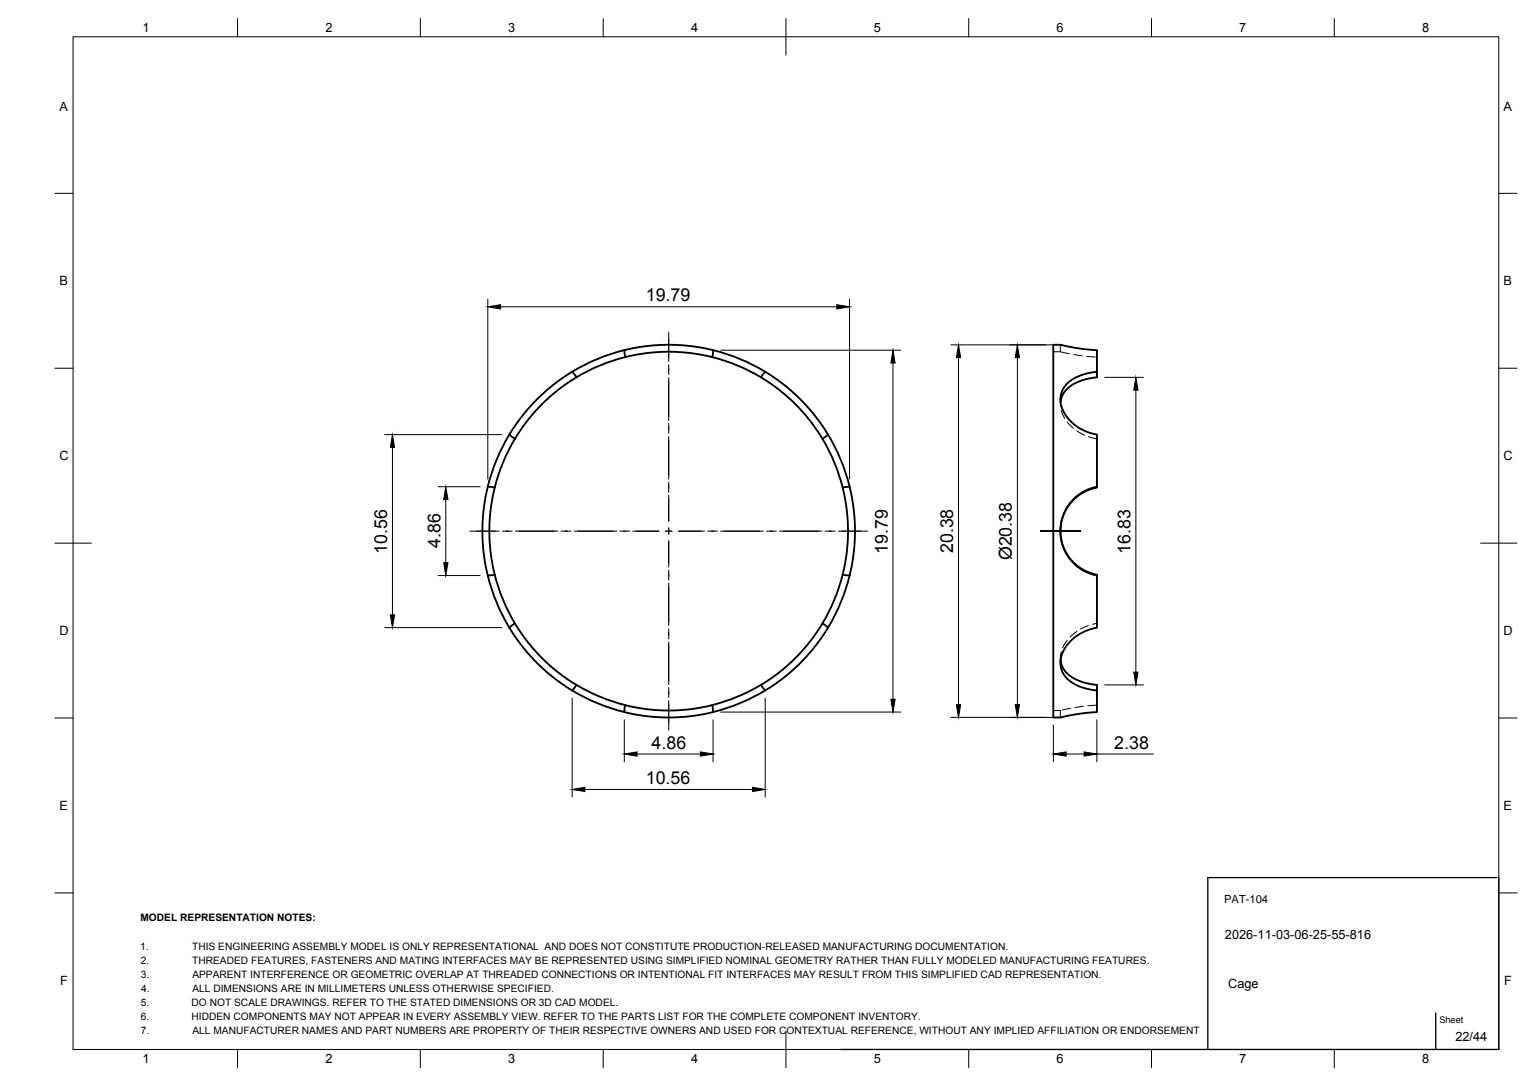
ISO-10303-21;
HEADER;
/* Generated by software containing ST-Developer
 * from STEP Tools, Inc. (www.steptools.com) 
 */

FILE_DESCRIPTION(
/* description */ ('Timing belt drive module 2 mm Pitch Timing 20T-40T'),

/* implementation_level */ '2;1');

FILE_NAME(
/* name */ 'Cage.step',
/* time_stamp */ '2026-10-28T03:25:12-07:00',
/* author */ (''),
/* organization */ (''),
/* preprocessor_version */ 'ST-DEVELOPER v20.2',
/* originating_system */ 'Autodesk Translation Framework v15.17.0.0',
/* authorisation */ '');

FILE_SCHEMA (('AUTOMOTIVE_DESIGN { 1 0 10303 214 3 1 1 }'));
ENDSEC;

DATA;
#10=MECHANICAL_DESIGN_GEOMETRIC_PRESENTATION_REPRESENTATION('',(#550),#17830);
#309=B_SPLINE_CURVE_WITH_KNOTS('',3,(#14805,#14806,#14807,#14808,#14809,
#14810,#14811,#14812,#14813,#14814,#14815,#14816,#14817,#14818,#14819,#14820,
#14821,#14822,#14823,#14824,#14825,#14826),.UNSPECIFIED.,.F.,.F.,(4,2,2,
2,2,2,2,2,2,2,4),(0.0473477652366656,0.126350602536658,0.189525903804987,
0.252701205073317,0.313298422430275,0.373895639787233,0.434492857144191,
0.495090074501149,0.558265375769478,0.621440677037807,0.7004435143378),
 .UNSPECIFIED.);
#310=B_SPLINE_CURVE_WITH_KNOTS('',3,(#14830,#14831,#14832,#14833,#14834,
#14835,#14836,#14837,#14838,#14839,#14840,#14841,#14842,#14843,#14844,#14845,
#14846,#14847,#14848,#14849,#14850,#14851),.UNSPECIFIED.,.F.,.F.,(4,2,2,
2,2,2,2,2,2,2,4),(0.0464897534940957,0.0852567806515119,0.170513561303024,
0.246687263103517,0.308657850341199,0.370628437578881,0.432599024816563,
0.494569612054245,0.570743313854739,0.656000094506251,0.694767121663666),
 .UNSPECIFIED.);
#311=B_SPLINE_CURVE_WITH_KNOTS('',3,(#14857,#14858,#14859,#14860,#14861,
#14862,#14863,#14864,#14865,#14866,#14867,#14868,#14869,#14870,#14871,#14872,
#14873,#14874,#14875,#14876,#14877,#14878),.UNSPECIFIED.,.F.,.F.,(4,2,2,
2,2,2,2,2,2,2,4),(0.0464897534940957,0.0852567806515118,0.170513561303024,
0.246687263103517,0.308657850341199,0.370628437578881,0.432599024816563,
0.494569612054245,0.570743313854738,0.65600009450625,0.694767121663666),
 .UNSPECIFIED.);
#312=B_SPLINE_CURVE_WITH_KNOTS('',3,(#14882,#14883,#14884,#14885,#14886,
#14887,#14888,#14889,#14890,#14891,#14892,#14893,#14894,#14895,#14896,#14897,
#14898,#14899,#14900,#14901,#14902,#14903),.UNSPECIFIED.,.F.,.F.,(4,2,2,
2,2,2,2,2,2,2,4),(0.0464897534940957,0.0852567806515119,0.170513561303024,
0.246687263103517,0.308657850341199,0.370628437578881,0.432599024816563,
0.494569612054245,0.570743313854739,0.656000094506251,0.694767121663666),
 .UNSPECIFIED.);
#313=B_SPLINE_CURVE_WITH_KNOTS('',3,(#14907,#14908,#14909,#14910,#14911,
#14912,#14913,#14914,#14915,#14916,#14917,#14918),.UNSPECIFIED.,.F.,.F.,
(4,2,2,2,2,4),(0.0464897534940957,0.0852567806515119,0.170513561303024,
0.246687263103517,0.308657850341199,0.370628437578881),.UNSPECIFIED.);
#314=B_SPLINE_CURVE_WITH_KNOTS('',3,(#14923,#14924,#14925,#14926,#14927,
#14928,#14929,#14930,#14931,#14932,#14933,#14934),.UNSPECIFIED.,.F.,.F.,
(4,2,2,2,2,4),(0.370628437578881,0.432599024816563,0.494569612054245,0.570743313854738,
0.65600009450625,0.694767121663666),.UNSPECIFIED.);
#315=B_SPLINE_CURVE_WITH_KNOTS('',3,(#14938,#14939,#14940,#14941,#14942,
#14943,#14944,#14945,#14946,#14947,#14948,#14949,#14950,#14951,#14952,#14953,
#14954,#14955,#14956,#14957,#14958,#14959),.UNSPECIFIED.,.F.,.F.,(4,2,2,
2,2,2,2,2,2,2,4),(0.0464897534940957,0.0852567806515121,0.170513561303024,
0.246687263103518,0.308657850341199,0.370628437578881,0.432599024816563,
0.494569612054245,0.570743313854738,0.65600009450625,0.694767121663666),
 .UNSPECIFIED.);
#316=B_SPLINE_CURVE_WITH_KNOTS('',3,(#14963,#14964,#14965,#14966,#14967,
#14968,#14969,#14970,#14971,#14972,#14973,#14974,#14975,#14976,#14977,#14978,
#14979,#14980,#14981,#14982,#14983,#14984),.UNSPECIFIED.,.F.,.F.,(4,2,2,
2,2,2,2,2,2,2,4),(0.0464897534940957,0.0852567806515119,0.170513561303024,
0.246687263103517,0.308657850341199,0.370628437578881,0.432599024816563,
0.494569612054245,0.570743313854738,0.65600009450625,0.694767121663667),
 .UNSPECIFIED.);
#317=B_SPLINE_CURVE_WITH_KNOTS('',3,(#14988,#14989,#14990,#14991,#14992,
#14993,#14994,#14995,#14996,#14997,#14998,#14999,#15000,#15001,#15002,#15003,
#15004,#15005,#15006,#15007,#15008,#15009),.UNSPECIFIED.,.F.,.F.,(4,2,2,
2,2,2,2,2,2,2,4),(0.0464897534940957,0.0852567806515119,0.170513561303024,
0.246687263103517,0.308657850341199,0.370628437578881,0.432599024816563,
0.494569612054245,0.570743313854738,0.65600009450625,0.694767121663666),
 .UNSPECIFIED.);
#318=B_SPLINE_CURVE_WITH_KNOTS('',3,(#15013,#15014,#15015,#15016,#15017,
#15018,#15019,#15020,#15021,#15022,#15023,#15024,#15025,#15026,#15027,#15028,
#15029,#15030,#15031,#15032,#15033,#15034),.UNSPECIFIED.,.F.,.F.,(4,2,2,
2,2,2,2,2,2,2,4),(0.0464897534940957,0.0852567806515119,0.170513561303024,
0.246687263103517,0.308657850341199,0.370628437578881,0.432599024816563,
0.494569612054245,0.570743313854739,0.656000094506251,0.694767121663667),
 .UNSPECIFIED.);
#319=B_SPLINE_CURVE_WITH_KNOTS('',3,(#15042,#15043,#15044,#15045,#15046,
#15047,#15048,#15049,#15050,#15051,#15052,#15053,#15054,#15055,#15056,#15057,
#15058,#15059,#15060,#15061,#15062,#15063),.UNSPECIFIED.,.F.,.F.,(4,2,2,
2,2,2,2,2,2,2,4),(0.0473477652366656,0.126350602536658,0.189525903804987,
0.252701205073316,0.313298422430274,0.373895639787232,0.434492857144191,
0.495090074501149,0.558265375769478,0.621440677037807,0.7004435143378),
 .UNSPECIFIED.);
#320=B_SPLINE_CURVE_WITH_KNOTS('',3,(#15071,#15072,#15073,#15074,#15075,
#15076,#15077,#15078,#15079,#15080,#15081,#15082,#15083,#15084,#15085,#15086,
#15087,#15088,#15089,#15090,#15091,#15092),.UNSPECIFIED.,.F.,.F.,(4,2,2,
2,2,2,2,2,2,2,4),(0.0473477652366656,0.126350602536658,0.189525903804987,
0.252701205073317,0.313298422430275,0.373895639787233,0.434492857144191,
0.495090074501149,0.558265375769478,0.621440677037807,0.7004435143378),
 .UNSPECIFIED.);
#321=B_SPLINE_CURVE_WITH_KNOTS('',3,(#15101,#15102,#15103,#15104,#15105,
#15106,#15107,#15108,#15109,#15110,#15111,#15112),.UNSPECIFIED.,.F.,.F.,
(4,2,2,2,2,4),(0.0473477652366656,0.126350602536658,0.189525903804987,0.252701205073316,
0.313298422430275,0.373895639787233),.UNSPECIFIED.);
#322=B_SPLINE_CURVE_WITH_KNOTS('',3,(#15114,#15115,#15116,#15117,#15118,
#15119,#15120,#15121,#15122,#15123,#15124,#15125),.UNSPECIFIED.,.F.,.F.,
(4,2,2,2,2,4),(0.373895639787233,0.434492857144191,0.495090074501149,0.558265375769478,
0.621440677037807,0.7004435143378),.UNSPECIFIED.);
#323=B_SPLINE_CURVE_WITH_KNOTS('',3,(#15132,#15133,#15134,#15135,#15136,
#15137,#15138,#15139,#15140,#15141,#15142,#15143,#15144,#15145,#15146,#15147,
#15148,#15149,#15150,#15151,#15152,#15153),.UNSPECIFIED.,.F.,.F.,(4,2,2,
2,2,2,2,2,2,2,4),(0.0473477652366656,0.126350602536658,0.189525903804987,
0.252701205073316,0.313298422430275,0.373895639787233,0.434492857144191,
0.495090074501149,0.558265375769478,0.621440677037807,0.7004435143378),
 .UNSPECIFIED.);
#324=B_SPLINE_CURVE_WITH_KNOTS('',3,(#15161,#15162,#15163,#15164,#15165,
#15166,#15167,#15168,#15169,#15170,#15171,#15172,#15173,#15174,#15175,#15176,
#15177,#15178,#15179,#15180,#15181,#15182),.UNSPECIFIED.,.F.,.F.,(4,2,2,
2,2,2,2,2,2,2,4),(0.0473477652366656,0.126350602536658,0.189525903804987,
0.252701205073317,0.313298422430275,0.373895639787233,0.434492857144191,
0.495090074501149,0.558265375769478,0.621440677037807,0.7004435143378),
 .UNSPECIFIED.);
#325=B_SPLINE_CURVE_WITH_KNOTS('',3,(#15190,#15191,#15192,#15193,#15194,
#15195,#15196,#15197,#15198,#15199,#15200,#15201,#15202,#15203,#15204,#15205,
#15206,#15207,#15208,#15209,#15210,#15211),.UNSPECIFIED.,.F.,.F.,(4,2,2,
2,2,2,2,2,2,2,4),(0.0473477652366656,0.126350602536658,0.189525903804987,
0.252701205073316,0.313298422430275,0.373895639787233,0.434492857144191,
0.495090074501149,0.558265375769478,0.621440677037807,0.7004435143378),
 .UNSPECIFIED.);
#326=B_SPLINE_CURVE_WITH_KNOTS('',3,(#15220,#15221,#15222,#15223,#15224,
#15225,#15226,#15227,#15228,#15229,#15230,#15231,#15232,#15233,#15234,#15235,
#15236,#15237,#15238,#15239,#15240,#15241),.UNSPECIFIED.,.F.,.F.,(4,2,2,
2,2,2,2,2,2,2,4),(0.0473477652366656,0.126350602536658,0.189525903804987,
0.252701205073317,0.313298422430275,0.373895639787233,0.434492857144191,
0.495090074501149,0.558265375769478,0.621440677037807,0.7004435143378),
 .UNSPECIFIED.);
#393=SPHERICAL_SURFACE('',#9935,0.247676);
#394=SPHERICAL_SURFACE('',#9951,0.247676);
#395=SPHERICAL_SURFACE('',#9956,0.247676);
#396=SPHERICAL_SURFACE('',#9961,0.247676);
#397=SPHERICAL_SURFACE('',#9966,0.247676);
#398=SPHERICAL_SURFACE('',#9971,0.247676);
#399=SPHERICAL_SURFACE('',#9976,0.247676);
#400=SPHERICAL_SURFACE('',#9984,0.247676);
#457=SHAPE_REPRESENTATION_RELATIONSHIP('SRR','None',#18028,#500);
#500=ADVANCED_BREP_SHAPE_REPRESENTATION('',(#608),#17803);
#550=STYLED_ITEM('',(#18317),#608);
#608=MANIFOLD_SOLID_BREP('Continuous crown cage',#9007);
#713=FACE_BOUND('',#1767,.T.);
#857=PLANE('',#9948);
#858=PLANE('',#9953);
#859=PLANE('',#9958);
#860=PLANE('',#9963);
#861=PLANE('',#9968);
#862=PLANE('',#9973);
#863=PLANE('',#9982);
#864=PLANE('',#9986);
#865=PLANE('',#9987);
#1152=FACE_OUTER_BOUND('',#1749,.T.);
#1153=FACE_OUTER_BOUND('',#1750,.T.);
#1154=FACE_OUTER_BOUND('',#1751,.T.);
#1155=FACE_OUTER_BOUND('',#1752,.T.);
#1156=FACE_OUTER_BOUND('',#1753,.T.);
#1157=FACE_OUTER_BOUND('',#1754,.T.);
#1158=FACE_OUTER_BOUND('',#1755,.T.);
#1159=FACE_OUTER_BOUND('',#1756,.T.);
#1160=FACE_OUTER_BOUND('',#1757,.T.);
#1161=FACE_OUTER_BOUND('',#1758,.T.);
#1162=FACE_OUTER_BOUND('',#1759,.T.);
#1163=FACE_OUTER_BOUND('',#1760,.T.);
#1164=FACE_OUTER_BOUND('',#1761,.T.);
#1165=FACE_OUTER_BOUND('',#1762,.T.);
#1166=FACE_OUTER_BOUND('',#1763,.T.);
#1167=FACE_OUTER_BOUND('',#1764,.T.);
#1168=FACE_OUTER_BOUND('',#1765,.T.);
#1169=FACE_OUTER_BOUND('',#1766,.T.);
#1170=FACE_OUTER_BOUND('',#1768,.T.);
#1749=EDGE_LOOP('',(#6621,#6622,#6623,#6624));
#1750=EDGE_LOOP('',(#6625,#6626,#6627,#6628,#6629,#6630,#6631,#6632,#6633,
#6634,#6635,#6636,#6637,#6638,#6639,#6640,#6641,#6642,#6643,#6644));
#1751=EDGE_LOOP('',(#6645,#6646,#6647,#6648));
#1752=EDGE_LOOP('',(#6649,#6650,#6651,#6652));
#1753=EDGE_LOOP('',(#6653,#6654,#6655,#6656));
#1754=EDGE_LOOP('',(#6657,#6658,#6659,#6660));
#1755=EDGE_LOOP('',(#6661,#6662,#6663,#6664));
#1756=EDGE_LOOP('',(#6665,#6666,#6667,#6668,#6669,#6670));
#1757=EDGE_LOOP('',(#6671,#6672,#6673,#6674));
#1758=EDGE_LOOP('',(#6675,#6676,#6677,#6678));
#1759=EDGE_LOOP('',(#6679,#6680,#6681,#6682));
#1760=EDGE_LOOP('',(#6683,#6684,#6685,#6686));
#1761=EDGE_LOOP('',(#6687,#6688,#6689,#6690));
#1762=EDGE_LOOP('',(#6691,#6692,#6693,#6694));
#1763=EDGE_LOOP('',(#6695,#6696,#6697,#6698,#6699,#6700,#6701,#6702,#6703,
#6704,#6705,#6706,#6707,#6708,#6709,#6710,#6711,#6712,#6713,#6714));
#1764=EDGE_LOOP('',(#6715,#6716,#6717,#6718));
#1765=EDGE_LOOP('',(#6719,#6720,#6721,#6722));
#1766=EDGE_LOOP('',(#6723));
#1767=EDGE_LOOP('',(#6724));
#1768=EDGE_LOOP('',(#6725,#6726,#6727,#6728));
#2346=CIRCLE('',#9936,0.243053047864041);
#2347=CIRCLE('',#9937,0.243053047864041);
#2348=CIRCLE('',#9939,1.019052);
#2349=CIRCLE('',#9940,1.019052);
#2350=CIRCLE('',#9941,1.019052);
#2351=CIRCLE('',#9942,1.019052);
#2352=CIRCLE('',#9943,1.019052);
#2353=CIRCLE('',#9944,1.019052);
#2354=CIRCLE('',#9945,1.019052);
#2355=CIRCLE('',#9946,1.019052);
#2356=CIRCLE('',#9947,1.019052);
#2357=CIRCLE('',#9949,0.980948);
#2358=CIRCLE('',#9950,0.243053047864041);
#2359=CIRCLE('',#9952,0.243053047864041);
#2360=CIRCLE('',#9954,0.980948);
#2361=CIRCLE('',#9955,0.243053047864041);
#2362=CIRCLE('',#9957,0.243053047864041);
#2363=CIRCLE('',#9959,0.980948);
#2364=CIRCLE('',#9960,0.243053047864041);
#2365=CIRCLE('',#9962,0.243053047864041);
#2366=CIRCLE('',#9964,0.980948);
#2367=CIRCLE('',#9965,0.243053047864041);
#2368=CIRCLE('',#9967,0.243053047864041);
#2369=CIRCLE('',#9969,0.980948);
#2370=CIRCLE('',#9970,0.243053047864041);
#2371=CIRCLE('',#9972,0.243053047864041);
#2372=CIRCLE('',#9974,0.980948);
#2373=CIRCLE('',#9975,0.243053047864041);
#2374=CIRCLE('',#9977,0.243053047864041);
#2375=CIRCLE('',#9979,0.980948);
#2376=CIRCLE('',#9980,0.980948);
#2377=CIRCLE('',#9981,0.980948);
#2378=CIRCLE('',#9983,0.243053047864041);
#2379=CIRCLE('',#9985,0.243053047864041);
#3008=LINE('',#14920,#3486);
#3009=LINE('',#15216,#3487);
#3486=VECTOR('',#11879,1.019052);
#3487=VECTOR('',#11956,0.980948);
#4038=VERTEX_POINT('',#14803);
#4039=VERTEX_POINT('',#14804);
#4040=VERTEX_POINT('',#14827);
#4041=VERTEX_POINT('',#14829);
#4042=VERTEX_POINT('',#14854);
#4043=VERTEX_POINT('',#14856);
#4044=VERTEX_POINT('',#14879);
#4045=VERTEX_POINT('',#14881);
#4046=VERTEX_POINT('',#14904);
#4047=VERTEX_POINT('',#14906);
#4048=VERTEX_POINT('',#14919);
#4049=VERTEX_POINT('',#14922);
#4050=VERTEX_POINT('',#14935);
#4051=VERTEX_POINT('',#14937);
#4052=VERTEX_POINT('',#14960);
#4053=VERTEX_POINT('',#14962);
#4054=VERTEX_POINT('',#14985);
#4055=VERTEX_POINT('',#14987);
#4056=VERTEX_POINT('',#15010);
#4057=VERTEX_POINT('',#15012);
#4058=VERTEX_POINT('',#15037);
#4059=VERTEX_POINT('',#15041);
#4060=VERTEX_POINT('',#15066);
#4061=VERTEX_POINT('',#15070);
#4062=VERTEX_POINT('',#15095);
#4063=VERTEX_POINT('',#15099);
#4064=VERTEX_POINT('',#15100);
#4065=VERTEX_POINT('',#15127);
#4066=VERTEX_POINT('',#15131);
#4067=VERTEX_POINT('',#15156);
#4068=VERTEX_POINT('',#15160);
#4069=VERTEX_POINT('',#15185);
#4070=VERTEX_POINT('',#15189);
#4071=VERTEX_POINT('',#15214);
#4072=VERTEX_POINT('',#15217);
#4073=VERTEX_POINT('',#15219);
#4993=EDGE_CURVE('',#4038,#4039,#309,.T.);
#4994=EDGE_CURVE('',#4040,#4038,#2346,.T.);
#4995=EDGE_CURVE('',#4041,#4040,#310,.T.);
#4996=EDGE_CURVE('',#4039,#4041,#2347,.T.);
#4997=EDGE_CURVE('',#4042,#4040,#2348,.T.);
#4998=EDGE_CURVE('',#4042,#4043,#311,.T.);
#4999=EDGE_CURVE('',#4044,#4043,#2349,.T.);
#5000=EDGE_CURVE('',#4044,#4045,#312,.T.);
#5001=EDGE_CURVE('',#4046,#4045,#2350,.T.);
#5002=EDGE_CURVE('',#4046,#4047,#313,.T.);
#5003=EDGE_CURVE('',#4047,#4048,#3008,.T.);
#5004=EDGE_CURVE('',#4048,#4048,#2351,.T.);
#5005=EDGE_CURVE('',#4047,#4049,#314,.T.);
#5006=EDGE_CURVE('',#4050,#4049,#2352,.T.);
#5007=EDGE_CURVE('',#4050,#4051,#315,.T.);
#5008=EDGE_CURVE('',#4052,#4051,#2353,.T.);
#5009=EDGE_CURVE('',#4052,#4053,#316,.T.);
#5010=EDGE_CURVE('',#4054,#4053,#2354,.T.);
#5011=EDGE_CURVE('',#4054,#4055,#317,.T.);
#5012=EDGE_CURVE('',#4056,#4055,#2355,.T.);
#5013=EDGE_CURVE('',#4056,#4057,#318,.T.);
#5014=EDGE_CURVE('',#4041,#4057,#2356,.T.);
#5015=EDGE_CURVE('',#4038,#4058,#2357,.T.);
#5016=EDGE_CURVE('',#4058,#4042,#2358,.T.);
#5017=EDGE_CURVE('',#4059,#4058,#319,.T.);
#5018=EDGE_CURVE('',#4043,#4059,#2359,.T.);
#5019=EDGE_CURVE('',#4059,#4060,#2360,.T.);
#5020=EDGE_CURVE('',#4060,#4044,#2361,.T.);
#5021=EDGE_CURVE('',#4061,#4060,#320,.T.);
#5022=EDGE_CURVE('',#4045,#4061,#2362,.T.);
#5023=EDGE_CURVE('',#4061,#4062,#2363,.T.);
#5024=EDGE_CURVE('',#4062,#4046,#2364,.T.);
#5025=EDGE_CURVE('',#4063,#4064,#321,.T.);
#5026=EDGE_CURVE('',#4049,#4063,#2365,.T.);
#5027=EDGE_CURVE('',#4064,#4062,#322,.T.);
#5028=EDGE_CURVE('',#4063,#4065,#2366,.T.);
#5029=EDGE_CURVE('',#4065,#4050,#2367,.T.);
#5030=EDGE_CURVE('',#4066,#4065,#323,.T.);
#5031=EDGE_CURVE('',#4051,#4066,#2368,.T.);
#5032=EDGE_CURVE('',#4066,#4067,#2369,.T.);
#5033=EDGE_CURVE('',#4067,#4052,#2370,.T.);
#5034=EDGE_CURVE('',#4068,#4067,#324,.T.);
#5035=EDGE_CURVE('',#4053,#4068,#2371,.T.);
#5036=EDGE_CURVE('',#4068,#4069,#2372,.T.);
#5037=EDGE_CURVE('',#4069,#4054,#2373,.T.);
#5038=EDGE_CURVE('',#4070,#4069,#325,.T.);
#5039=EDGE_CURVE('',#4055,#4070,#2374,.T.);
#5040=EDGE_CURVE('',#4071,#4071,#2375,.T.);
#5041=EDGE_CURVE('',#4071,#4064,#3009,.T.);
#5042=EDGE_CURVE('',#4072,#4039,#2376,.T.);
#5043=EDGE_CURVE('',#4072,#4073,#326,.T.);
#5044=EDGE_CURVE('',#4070,#4073,#2377,.T.);
#5045=EDGE_CURVE('',#4057,#4072,#2378,.T.);
#5046=EDGE_CURVE('',#4073,#4056,#2379,.T.);
#6621=ORIENTED_EDGE('',*,*,#4993,.F.);
#6622=ORIENTED_EDGE('',*,*,#4994,.F.);
#6623=ORIENTED_EDGE('',*,*,#4995,.F.);
#6624=ORIENTED_EDGE('',*,*,#4996,.F.);
#6625=ORIENTED_EDGE('',*,*,#4995,.T.);
#6626=ORIENTED_EDGE('',*,*,#4997,.F.);
#6627=ORIENTED_EDGE('',*,*,#4998,.T.);
#6628=ORIENTED_EDGE('',*,*,#4999,.F.);
#6629=ORIENTED_EDGE('',*,*,#5000,.T.);
#6630=ORIENTED_EDGE('',*,*,#5001,.F.);
#6631=ORIENTED_EDGE('',*,*,#5002,.T.);
#6632=ORIENTED_EDGE('',*,*,#5003,.T.);
#6633=ORIENTED_EDGE('',*,*,#5004,.F.);
#6634=ORIENTED_EDGE('',*,*,#5003,.F.);
#6635=ORIENTED_EDGE('',*,*,#5005,.T.);
#6636=ORIENTED_EDGE('',*,*,#5006,.F.);
#6637=ORIENTED_EDGE('',*,*,#5007,.T.);
#6638=ORIENTED_EDGE('',*,*,#5008,.F.);
#6639=ORIENTED_EDGE('',*,*,#5009,.T.);
#6640=ORIENTED_EDGE('',*,*,#5010,.F.);
#6641=ORIENTED_EDGE('',*,*,#5011,.T.);
#6642=ORIENTED_EDGE('',*,*,#5012,.F.);
#6643=ORIENTED_EDGE('',*,*,#5013,.T.);
#6644=ORIENTED_EDGE('',*,*,#5014,.F.);
#6645=ORIENTED_EDGE('',*,*,#4994,.T.);
#6646=ORIENTED_EDGE('',*,*,#5015,.T.);
#6647=ORIENTED_EDGE('',*,*,#5016,.T.);
#6648=ORIENTED_EDGE('',*,*,#4997,.T.);
#6649=ORIENTED_EDGE('',*,*,#5017,.F.);
#6650=ORIENTED_EDGE('',*,*,#5018,.F.);
#6651=ORIENTED_EDGE('',*,*,#4998,.F.);
#6652=ORIENTED_EDGE('',*,*,#5016,.F.);
#6653=ORIENTED_EDGE('',*,*,#5018,.T.);
#6654=ORIENTED_EDGE('',*,*,#5019,.T.);
#6655=ORIENTED_EDGE('',*,*,#5020,.T.);
#6656=ORIENTED_EDGE('',*,*,#4999,.T.);
#6657=ORIENTED_EDGE('',*,*,#5021,.F.);
#6658=ORIENTED_EDGE('',*,*,#5022,.F.);
#6659=ORIENTED_EDGE('',*,*,#5000,.F.);
#6660=ORIENTED_EDGE('',*,*,#5020,.F.);
#6661=ORIENTED_EDGE('',*,*,#5022,.T.);
#6662=ORIENTED_EDGE('',*,*,#5023,.T.);
#6663=ORIENTED_EDGE('',*,*,#5024,.T.);
#6664=ORIENTED_EDGE('',*,*,#5001,.T.);
#6665=ORIENTED_EDGE('',*,*,#5025,.F.);
#6666=ORIENTED_EDGE('',*,*,#5026,.F.);
#6667=ORIENTED_EDGE('',*,*,#5005,.F.);
#6668=ORIENTED_EDGE('',*,*,#5002,.F.);
#6669=ORIENTED_EDGE('',*,*,#5024,.F.);
#6670=ORIENTED_EDGE('',*,*,#5027,.F.);
#6671=ORIENTED_EDGE('',*,*,#5026,.T.);
#6672=ORIENTED_EDGE('',*,*,#5028,.T.);
#6673=ORIENTED_EDGE('',*,*,#5029,.T.);
#6674=ORIENTED_EDGE('',*,*,#5006,.T.);
#6675=ORIENTED_EDGE('',*,*,#5030,.F.);
#6676=ORIENTED_EDGE('',*,*,#5031,.F.);
#6677=ORIENTED_EDGE('',*,*,#5007,.F.);
#6678=ORIENTED_EDGE('',*,*,#5029,.F.);
#6679=ORIENTED_EDGE('',*,*,#5031,.T.);
#6680=ORIENTED_EDGE('',*,*,#5032,.T.);
#6681=ORIENTED_EDGE('',*,*,#5033,.T.);
#6682=ORIENTED_EDGE('',*,*,#5008,.T.);
#6683=ORIENTED_EDGE('',*,*,#5034,.F.);
#6684=ORIENTED_EDGE('',*,*,#5035,.F.);
#6685=ORIENTED_EDGE('',*,*,#5009,.F.);
#6686=ORIENTED_EDGE('',*,*,#5033,.F.);
#6687=ORIENTED_EDGE('',*,*,#5035,.T.);
#6688=ORIENTED_EDGE('',*,*,#5036,.T.);
#6689=ORIENTED_EDGE('',*,*,#5037,.T.);
#6690=ORIENTED_EDGE('',*,*,#5010,.T.);
#6691=ORIENTED_EDGE('',*,*,#5011,.F.);
#6692=ORIENTED_EDGE('',*,*,#5037,.F.);
#6693=ORIENTED_EDGE('',*,*,#5038,.F.);
#6694=ORIENTED_EDGE('',*,*,#5039,.F.);
#6695=ORIENTED_EDGE('',*,*,#5040,.F.);
#6696=ORIENTED_EDGE('',*,*,#5041,.T.);
#6697=ORIENTED_EDGE('',*,*,#5027,.T.);
#6698=ORIENTED_EDGE('',*,*,#5023,.F.);
#6699=ORIENTED_EDGE('',*,*,#5021,.T.);
#6700=ORIENTED_EDGE('',*,*,#5019,.F.);
#6701=ORIENTED_EDGE('',*,*,#5017,.T.);
#6702=ORIENTED_EDGE('',*,*,#5015,.F.);
#6703=ORIENTED_EDGE('',*,*,#4993,.T.);
#6704=ORIENTED_EDGE('',*,*,#5042,.F.);
#6705=ORIENTED_EDGE('',*,*,#5043,.T.);
#6706=ORIENTED_EDGE('',*,*,#5044,.F.);
#6707=ORIENTED_EDGE('',*,*,#5038,.T.);
#6708=ORIENTED_EDGE('',*,*,#5036,.F.);
#6709=ORIENTED_EDGE('',*,*,#5034,.T.);
#6710=ORIENTED_EDGE('',*,*,#5032,.F.);
#6711=ORIENTED_EDGE('',*,*,#5030,.T.);
#6712=ORIENTED_EDGE('',*,*,#5028,.F.);
#6713=ORIENTED_EDGE('',*,*,#5025,.T.);
#6714=ORIENTED_EDGE('',*,*,#5041,.F.);
#6715=ORIENTED_EDGE('',*,*,#4996,.T.);
#6716=ORIENTED_EDGE('',*,*,#5014,.T.);
#6717=ORIENTED_EDGE('',*,*,#5045,.T.);
#6718=ORIENTED_EDGE('',*,*,#5042,.T.);
#6719=ORIENTED_EDGE('',*,*,#5013,.F.);
#6720=ORIENTED_EDGE('',*,*,#5046,.F.);
#6721=ORIENTED_EDGE('',*,*,#5043,.F.);
#6722=ORIENTED_EDGE('',*,*,#5045,.F.);
#6723=ORIENTED_EDGE('',*,*,#5004,.T.);
#6724=ORIENTED_EDGE('',*,*,#5040,.T.);
#6725=ORIENTED_EDGE('',*,*,#5039,.T.);
#6726=ORIENTED_EDGE('',*,*,#5044,.T.);
#6727=ORIENTED_EDGE('',*,*,#5046,.T.);
#6728=ORIENTED_EDGE('',*,*,#5012,.T.);
#8273=CYLINDRICAL_SURFACE('',#9938,1.019052);
#8274=CYLINDRICAL_SURFACE('',#9978,0.980948);
#8650=ADVANCED_FACE('',(#1152),#393,.F.);
#8651=ADVANCED_FACE('',(#1153),#8273,.T.);
#8652=ADVANCED_FACE('',(#1154),#857,.T.);
#8653=ADVANCED_FACE('',(#1155),#394,.F.);
#8654=ADVANCED_FACE('',(#1156),#858,.T.);
#8655=ADVANCED_FACE('',(#1157),#395,.F.);
#8656=ADVANCED_FACE('',(#1158),#859,.T.);
#8657=ADVANCED_FACE('',(#1159),#396,.F.);
#8658=ADVANCED_FACE('',(#1160),#860,.T.);
#8659=ADVANCED_FACE('',(#1161),#397,.F.);
#8660=ADVANCED_FACE('',(#1162),#861,.T.);
#8661=ADVANCED_FACE('',(#1163),#398,.F.);
#8662=ADVANCED_FACE('',(#1164),#862,.T.);
#8663=ADVANCED_FACE('',(#1165),#399,.F.);
#8664=ADVANCED_FACE('',(#1166),#8274,.F.);
#8665=ADVANCED_FACE('',(#1167),#863,.T.);
#8666=ADVANCED_FACE('',(#1168),#400,.F.);
#8667=ADVANCED_FACE('',(#1169,#713),#864,.T.);
#8668=ADVANCED_FACE('',(#1170),#865,.T.);
#9007=CLOSED_SHELL('',(#8650,#8651,#8652,#8653,#8654,#8655,#8656,#8657,
#8658,#8659,#8660,#8661,#8662,#8663,#8664,#8665,#8666,#8667,#8668));
#9934=AXIS2_PLACEMENT_3D('',#14801,#11863,#11864);
#9935=AXIS2_PLACEMENT_3D('',#14802,#11865,#11866);
#9936=AXIS2_PLACEMENT_3D('',#14828,#11867,#11868);
#9937=AXIS2_PLACEMENT_3D('',#14852,#11869,#11870);
#9938=AXIS2_PLACEMENT_3D('',#14853,#11871,#11872);
#9939=AXIS2_PLACEMENT_3D('',#14855,#11873,#11874);
#9940=AXIS2_PLACEMENT_3D('',#14880,#11875,#11876);
#9941=AXIS2_PLACEMENT_3D('',#14905,#11877,#11878);
#9942=AXIS2_PLACEMENT_3D('',#14921,#11880,#11881);
#9943=AXIS2_PLACEMENT_3D('',#14936,#11882,#11883);
#9944=AXIS2_PLACEMENT_3D('',#14961,#11884,#11885);
#9945=AXIS2_PLACEMENT_3D('',#14986,#11886,#11887);
#9946=AXIS2_PLACEMENT_3D('',#15011,#11888,#11889);
#9947=AXIS2_PLACEMENT_3D('',#15035,#11890,#11891);
#9948=AXIS2_PLACEMENT_3D('',#15036,#11892,#11893);
#9949=AXIS2_PLACEMENT_3D('',#15038,#11894,#11895);
#9950=AXIS2_PLACEMENT_3D('',#15039,#11896,#11897);
#9951=AXIS2_PLACEMENT_3D('',#15040,#11898,#11899);
#9952=AXIS2_PLACEMENT_3D('',#15064,#11900,#11901);
#9953=AXIS2_PLACEMENT_3D('',#15065,#11902,#11903);
#9954=AXIS2_PLACEMENT_3D('',#15067,#11904,#11905);
#9955=AXIS2_PLACEMENT_3D('',#15068,#11906,#11907);
#9956=AXIS2_PLACEMENT_3D('',#15069,#11908,#11909);
#9957=AXIS2_PLACEMENT_3D('',#15093,#11910,#11911);
#9958=AXIS2_PLACEMENT_3D('',#15094,#11912,#11913);
#9959=AXIS2_PLACEMENT_3D('',#15096,#11914,#11915);
#9960=AXIS2_PLACEMENT_3D('',#15097,#11916,#11917);
#9961=AXIS2_PLACEMENT_3D('',#15098,#11918,#11919);
#9962=AXIS2_PLACEMENT_3D('',#15113,#11920,#11921);
#9963=AXIS2_PLACEMENT_3D('',#15126,#11922,#11923);
#9964=AXIS2_PLACEMENT_3D('',#15128,#11924,#11925);
#9965=AXIS2_PLACEMENT_3D('',#15129,#11926,#11927);
#9966=AXIS2_PLACEMENT_3D('',#15130,#11928,#11929);
#9967=AXIS2_PLACEMENT_3D('',#15154,#11930,#11931);
#9968=AXIS2_PLACEMENT_3D('',#15155,#11932,#11933);
#9969=AXIS2_PLACEMENT_3D('',#15157,#11934,#11935);
#9970=AXIS2_PLACEMENT_3D('',#15158,#11936,#11937);
#9971=AXIS2_PLACEMENT_3D('',#15159,#11938,#11939);
#9972=AXIS2_PLACEMENT_3D('',#15183,#11940,#11941);
#9973=AXIS2_PLACEMENT_3D('',#15184,#11942,#11943);
#9974=AXIS2_PLACEMENT_3D('',#15186,#11944,#11945);
#9975=AXIS2_PLACEMENT_3D('',#15187,#11946,#11947);
#9976=AXIS2_PLACEMENT_3D('',#15188,#11948,#11949);
#9977=AXIS2_PLACEMENT_3D('',#15212,#11950,#11951);
#9978=AXIS2_PLACEMENT_3D('',#15213,#11952,#11953);
#9979=AXIS2_PLACEMENT_3D('',#15215,#11954,#11955);
#9980=AXIS2_PLACEMENT_3D('',#15218,#11957,#11958);
#9981=AXIS2_PLACEMENT_3D('',#15242,#11959,#11960);
#9982=AXIS2_PLACEMENT_3D('',#15243,#11961,#11962);
#9983=AXIS2_PLACEMENT_3D('',#15244,#11963,#11964);
#9984=AXIS2_PLACEMENT_3D('',#15245,#11965,#11966);
#9985=AXIS2_PLACEMENT_3D('',#15246,#11967,#11968);
#9986=AXIS2_PLACEMENT_3D('',#15247,#11969,#11970);
#9987=AXIS2_PLACEMENT_3D('',#15248,#11971,#11972);
#11863=DIRECTION('axis',(0.,0.,1.));
#11864=DIRECTION('refdir',(1.,0.,0.));
#11865=DIRECTION('center_axis',(0.,0.,1.));
#11866=DIRECTION('ref_axis',(1.,0.,0.));
#11867=DIRECTION('center_axis',(0.,-1.,0.));
#11868=DIRECTION('ref_axis',(0.,0.,-1.));
#11869=DIRECTION('center_axis',(0.,-1.,0.));
#11870=DIRECTION('ref_axis',(0.,0.,-1.));
#11871=DIRECTION('center_axis',(0.,1.,0.));
#11872=DIRECTION('ref_axis',(1.,0.,0.));
#11873=DIRECTION('center_axis',(0.,1.,0.));
#11874=DIRECTION('ref_axis',(1.,0.,0.));
#11875=DIRECTION('center_axis',(0.,1.,0.));
#11876=DIRECTION('ref_axis',(1.,0.,0.));
#11877=DIRECTION('center_axis',(0.,1.,0.));
#11878=DIRECTION('ref_axis',(1.,0.,0.));
#11879=DIRECTION('',(0.,-1.,0.));
#11880=DIRECTION('center_axis',(0.,-1.,0.));
#11881=DIRECTION('ref_axis',(1.,0.,0.));
#11882=DIRECTION('center_axis',(0.,1.,0.));
#11883=DIRECTION('ref_axis',(1.,0.,0.));
#11884=DIRECTION('center_axis',(0.,1.,0.));
#11885=DIRECTION('ref_axis',(1.,0.,0.));
#11886=DIRECTION('center_axis',(0.,1.,0.));
#11887=DIRECTION('ref_axis',(1.,0.,0.));
#11888=DIRECTION('center_axis',(0.,1.,0.));
#11889=DIRECTION('ref_axis',(1.,0.,0.));
#11890=DIRECTION('center_axis',(0.,1.,0.));
#11891=DIRECTION('ref_axis',(1.,0.,0.));
#11892=DIRECTION('center_axis',(0.,1.,0.));
#11893=DIRECTION('ref_axis',(1.,0.,0.));
#11894=DIRECTION('center_axis',(0.,-1.,0.));
#11895=DIRECTION('ref_axis',(1.,0.,0.));
#11896=DIRECTION('center_axis',(0.,-1.,0.));
#11897=DIRECTION('ref_axis',(0.,0.,-1.));
#11898=DIRECTION('center_axis',(6.12323399573677E-17,0.,1.));
#11899=DIRECTION('ref_axis',(1.,0.,0.));
#11900=DIRECTION('center_axis',(0.,-1.,0.));
#11901=DIRECTION('ref_axis',(0.,0.,-1.));
#11902=DIRECTION('center_axis',(0.,1.,0.));
#11903=DIRECTION('ref_axis',(1.,0.,0.));
#11904=DIRECTION('center_axis',(0.,-1.,0.));
#11905=DIRECTION('ref_axis',(1.,0.,0.));
#11906=DIRECTION('center_axis',(0.,-1.,0.));
#11907=DIRECTION('ref_axis',(0.,0.,-1.));
#11908=DIRECTION('center_axis',(0.,0.,1.));
#11909=DIRECTION('ref_axis',(1.,0.,0.));
#11910=DIRECTION('center_axis',(0.,-1.,0.));
#11911=DIRECTION('ref_axis',(0.,0.,-1.));
#11912=DIRECTION('center_axis',(0.,1.,0.));
#11913=DIRECTION('ref_axis',(1.,0.,0.));
#11914=DIRECTION('center_axis',(0.,-1.,0.));
#11915=DIRECTION('ref_axis',(1.,0.,0.));
#11916=DIRECTION('center_axis',(0.,-1.,0.));
#11917=DIRECTION('ref_axis',(0.,0.,-1.));
#11918=DIRECTION('center_axis',(0.,0.,1.));
#11919=DIRECTION('ref_axis',(1.,0.,0.));
#11920=DIRECTION('center_axis',(0.,-1.,0.));
#11921=DIRECTION('ref_axis',(0.,0.,-1.));
#11922=DIRECTION('center_axis',(0.,1.,0.));
#11923=DIRECTION('ref_axis',(1.,0.,0.));
#11924=DIRECTION('center_axis',(0.,-1.,0.));
#11925=DIRECTION('ref_axis',(1.,0.,0.));
#11926=DIRECTION('center_axis',(0.,-1.,0.));
#11927=DIRECTION('ref_axis',(0.,0.,-1.));
#11928=DIRECTION('center_axis',(0.,0.,1.));
#11929=DIRECTION('ref_axis',(1.,0.,0.));
#11930=DIRECTION('center_axis',(0.,-1.,0.));
#11931=DIRECTION('ref_axis',(0.,0.,-1.));
#11932=DIRECTION('center_axis',(0.,1.,0.));
#11933=DIRECTION('ref_axis',(1.,0.,0.));
#11934=DIRECTION('center_axis',(0.,-1.,0.));
#11935=DIRECTION('ref_axis',(1.,0.,0.));
#11936=DIRECTION('center_axis',(0.,-1.,0.));
#11937=DIRECTION('ref_axis',(0.,0.,-1.));
#11938=DIRECTION('center_axis',(6.12323399573676E-17,0.,1.));
#11939=DIRECTION('ref_axis',(1.,0.,0.));
#11940=DIRECTION('center_axis',(0.,-1.,0.));
#11941=DIRECTION('ref_axis',(0.,0.,-1.));
#11942=DIRECTION('center_axis',(0.,1.,0.));
#11943=DIRECTION('ref_axis',(1.,0.,0.));
#11944=DIRECTION('center_axis',(0.,-1.,0.));
#11945=DIRECTION('ref_axis',(1.,0.,0.));
#11946=DIRECTION('center_axis',(0.,-1.,0.));
#11947=DIRECTION('ref_axis',(0.,0.,-1.));
#11948=DIRECTION('center_axis',(0.,0.,1.));
#11949=DIRECTION('ref_axis',(1.,0.,0.));
#11950=DIRECTION('center_axis',(0.,-1.,0.));
#11951=DIRECTION('ref_axis',(0.,0.,-1.));
#11952=DIRECTION('center_axis',(0.,1.,0.));
#11953=DIRECTION('ref_axis',(1.,0.,0.));
#11954=DIRECTION('center_axis',(0.,1.,0.));
#11955=DIRECTION('ref_axis',(1.,0.,0.));
#11956=DIRECTION('',(0.,1.,0.));
#11957=DIRECTION('center_axis',(0.,-1.,0.));
#11958=DIRECTION('ref_axis',(1.,0.,0.));
#11959=DIRECTION('center_axis',(0.,-1.,0.));
#11960=DIRECTION('ref_axis',(1.,0.,0.));
#11961=DIRECTION('center_axis',(0.,1.,0.));
#11962=DIRECTION('ref_axis',(1.,0.,0.));
#11963=DIRECTION('center_axis',(0.,-1.,0.));
#11964=DIRECTION('ref_axis',(0.,0.,-1.));
#11965=DIRECTION('center_axis',(0.,0.,1.));
#11966=DIRECTION('ref_axis',(1.,0.,0.));
#11967=DIRECTION('center_axis',(0.,-1.,0.));
#11968=DIRECTION('ref_axis',(0.,0.,-1.));
#11969=DIRECTION('center_axis',(0.,-1.,0.));
#11970=DIRECTION('ref_axis',(-1.,0.,0.));
#11971=DIRECTION('center_axis',(0.,1.,0.));
#11972=DIRECTION('ref_axis',(1.,0.,0.));
#14801=CARTESIAN_POINT('',(0.,0.,0.));
#14802=CARTESIAN_POINT('Origin',(0.707106781186547,0.,0.707106781186548));
#14803=CARTESIAN_POINT('',(0.504455939115715,-0.04763,0.841298510752802));
#14804=CARTESIAN_POINT('',(0.841298510752802,-0.04763,0.504455939115715));
#14805=CARTESIAN_POINT('Ctrl Pts',(0.504455939115715,-0.04763,0.841298510752802));
#14806=CARTESIAN_POINT('Ctrl Pts',(0.508899795931835,-0.0740444353928835,
0.838633903678357));
#14807=CARTESIAN_POINT('Ctrl Pts',(0.517157748491652,-0.0999305678883309,
0.833661031856294));
#14808=CARTESIAN_POINT('Ctrl Pts',(0.537715343527944,-0.142345102874864,
0.820511285096538));
#14809=CARTESIAN_POINT('Ctrl Pts',(0.548874290046456,-0.159766064500479,
0.813159949759));
#14810=CARTESIAN_POINT('Ctrl Pts',(0.573915184558107,-0.190326085855194,
0.795684265985089));
#14811=CARTESIAN_POINT('Ctrl Pts',(0.587792702767295,-0.203463743702801,
0.78555112003688));
#14812=CARTESIAN_POINT('Ctrl Pts',(0.615966552324775,-0.224161999508995,
0.763642258217233));
#14813=CARTESIAN_POINT('Ctrl Pts',(0.631684198665438,-0.232861760990032,
0.750785745543687));
#14814=CARTESIAN_POINT('Ctrl Pts',(0.663382628119203,-0.244251601209411,
0.722929908501543));
#14815=CARTESIAN_POINT('Ctrl Pts',(0.679352081686668,-0.246942143572133,
0.707917883896095));
#14816=CARTESIAN_POINT('Ctrl Pts',(0.707917883896095,-0.246942143572133,
0.679352081686668));
#14817=CARTESIAN_POINT('Ctrl Pts',(0.722929908501543,-0.244251601209411,
0.663382628119203));
#14818=CARTESIAN_POINT('Ctrl Pts',(0.750785745543687,-0.232861760990032,
0.631684198665439));
#14819=CARTESIAN_POINT('Ctrl Pts',(0.763642258217232,-0.224161999508995,
0.615966552324775));
#14820=CARTESIAN_POINT('Ctrl Pts',(0.78555112003688,-0.203463743702801,
0.587792702767295));
#14821=CARTESIAN_POINT('Ctrl Pts',(0.795684265985088,-0.190326085855194,
0.573915184558108));
#14822=CARTESIAN_POINT('Ctrl Pts',(0.813159949759,-0.15976606450048,0.548874290046456));
#14823=CARTESIAN_POINT('Ctrl Pts',(0.820511285096538,-0.142345102874864,
0.537715343527944));
#14824=CARTESIAN_POINT('Ctrl Pts',(0.833661031856294,-0.099930567888331,
0.517157748491653));
#14825=CARTESIAN_POINT('Ctrl Pts',(0.838633903678357,-0.0740444353928835,
0.508899795931835));
#14826=CARTESIAN_POINT('Ctrl Pts',(0.841298510752801,-0.0476299999999999,
0.504455939115715));
#14827=CARTESIAN_POINT('',(0.528110872004958,-0.04763,0.871530771444223));
#14828=CARTESIAN_POINT('Origin',(0.707106781186547,-0.04763,0.707106781186548));
#14829=CARTESIAN_POINT('',(0.871530771444223,-0.04763,0.528110872004959));
#14830=CARTESIAN_POINT('Ctrl Pts',(0.871530771444223,-0.0476300000000001,
0.528110872004958));
#14831=CARTESIAN_POINT('Ctrl Pts',(0.87014664509073,-0.0609922781173483,
0.530395067942936));
#14832=CARTESIAN_POINT('Ctrl Pts',(0.868149331745851,-0.0742967091364493,
0.533674141594226));
#14833=CARTESIAN_POINT('Ctrl Pts',(0.85981294420286,-0.115492077056649,
0.54708917182331));
#14834=CARTESIAN_POINT('Ctrl Pts',(0.850993704737257,-0.141695629206859,
0.560922177770136));
#14835=CARTESIAN_POINT('Ctrl Pts',(0.830754510485543,-0.181890537957859,
0.590422647829571));
#14836=CARTESIAN_POINT('Ctrl Pts',(0.816896541396381,-0.201072148666545,
0.609616703125488));
#14837=CARTESIAN_POINT('Ctrl Pts',(0.792310597819928,-0.223955109275652,
0.641117951819998));
#14838=CARTESIAN_POINT('Ctrl Pts',(0.779109323683612,-0.232742381310829,
0.657208095763053));
#14839=CARTESIAN_POINT('Ctrl Pts',(0.750552691816206,-0.244234834628584,
0.68964083160521));
#14840=CARTESIAN_POINT('Ctrl Pts',(0.735185187071673,-0.246942143572133,
0.705971972091755));
#14841=CARTESIAN_POINT('Ctrl Pts',(0.705971972091754,-0.246942143572133,
0.735185187071673));
#14842=CARTESIAN_POINT('Ctrl Pts',(0.689640831605209,-0.244234834628584,
0.750552691816206));
#14843=CARTESIAN_POINT('Ctrl Pts',(0.657208095763052,-0.232742381310829,
0.779109323683612));
#14844=CARTESIAN_POINT('Ctrl Pts',(0.641117951819998,-0.223955109275652,
0.792310597819928));
#14845=CARTESIAN_POINT('Ctrl Pts',(0.609616703125487,-0.201072148666545,
0.816896541396382));
#14846=CARTESIAN_POINT('Ctrl Pts',(0.590422647829571,-0.181890537957858,
0.830754510485544));
#14847=CARTESIAN_POINT('Ctrl Pts',(0.560922177770135,-0.141695629206858,
0.850993704737257));
#14848=CARTESIAN_POINT('Ctrl Pts',(0.547089171823309,-0.115492077056649,
0.859812944202861));
#14849=CARTESIAN_POINT('Ctrl Pts',(0.533674141594226,-0.0742967091364491,
0.868149331745852));
#14850=CARTESIAN_POINT('Ctrl Pts',(0.530395067942936,-0.0609922781173483,
0.870146645090731));
#14851=CARTESIAN_POINT('Ctrl Pts',(0.528110872004958,-0.0476300000000001,
0.871530771444223));
#14852=CARTESIAN_POINT('Origin',(0.707106781186547,-0.04763,0.707106781186548));
#14853=CARTESIAN_POINT('Origin',(0.,-0.166705,0.));
#14854=CARTESIAN_POINT('',(0.242834539687906,-0.04763,0.989696097314));
#14855=CARTESIAN_POINT('Origin',(0.,-0.04763,0.));
#14856=CARTESIAN_POINT('',(-0.242834539687907,-0.04763,0.989696097314));
#14857=CARTESIAN_POINT('Ctrl Pts',(0.242834539687906,-0.04763,0.989696097314));
#14858=CARTESIAN_POINT('Ctrl Pts',(0.24024064412003,-0.0609922781173483,
0.990332542620729));
#14859=CARTESIAN_POINT('Ctrl Pts',(0.236509675094874,-0.0742967091364492,
0.991238884025248));
#14860=CARTESIAN_POINT('Ctrl Pts',(0.221129100087819,-0.115492077056649,
0.994830026707808));
#14861=CARTESIAN_POINT('Ctrl Pts',(0.205111543747588,-0.141695629206859,
0.998375294985966));
#14862=CARTESIAN_POINT('Ctrl Pts',(0.169940289819232,-0.181890537957859,
1.00492400591205));
#14863=CARTESIAN_POINT('Ctrl Pts',(0.1465689792446,-0.201072148666545,1.00869718865384));
#14864=CARTESIAN_POINT('Ctrl Pts',(0.106909345252087,-0.223955109275652,
1.01358704779679));
#14865=CARTESIAN_POINT('Ctrl Pts',(0.0861971848975941,-0.232742381310829,
1.0156297872271));
#14866=CARTESIAN_POINT('Ctrl Pts',(0.0430711894098822,-0.244234834628584,
1.01837060663223));
#14867=CARTESIAN_POINT('Ctrl Pts',(0.0206568624125605,-0.246942143572133,
1.019052));
#14868=CARTESIAN_POINT('Ctrl Pts',(-0.0206568624125608,-0.246942143572133,
1.019052));
#14869=CARTESIAN_POINT('Ctrl Pts',(-0.0430711894098825,-0.244234834628584,
1.01837060663223));
#14870=CARTESIAN_POINT('Ctrl Pts',(-0.0861971848975943,-0.232742381310829,
1.0156297872271));
#14871=CARTESIAN_POINT('Ctrl Pts',(-0.106909345252088,-0.223955109275652,
1.01358704779679));
#14872=CARTESIAN_POINT('Ctrl Pts',(-0.1465689792446,-0.201072148666545,
1.00869718865384));
#14873=CARTESIAN_POINT('Ctrl Pts',(-0.169940289819232,-0.181890537957859,
1.00492400591205));
#14874=CARTESIAN_POINT('Ctrl Pts',(-0.205111543747588,-0.141695629206859,
0.998375294985966));
#14875=CARTESIAN_POINT('Ctrl Pts',(-0.221129100087819,-0.115492077056649,
0.994830026707808));
#14876=CARTESIAN_POINT('Ctrl Pts',(-0.236509675094875,-0.0742967091364493,
0.991238884025248));
#14877=CARTESIAN_POINT('Ctrl Pts',(-0.24024064412003,-0.0609922781173483,
0.990332542620729));
#14878=CARTESIAN_POINT('Ctrl Pts',(-0.242834539687907,-0.04763,0.989696097314));
#14879=CARTESIAN_POINT('',(-0.528110872004959,-0.04763,0.871530771444223));
#14880=CARTESIAN_POINT('Origin',(0.,-0.04763,0.));
#14881=CARTESIAN_POINT('',(-0.871530771444223,-0.04763,0.528110872004958));
#14882=CARTESIAN_POINT('Ctrl Pts',(-0.528110872004958,-0.0476300000000001,
0.871530771444223));
#14883=CARTESIAN_POINT('Ctrl Pts',(-0.530395067942936,-0.0609922781173484,
0.87014664509073));
#14884=CARTESIAN_POINT('Ctrl Pts',(-0.533674141594226,-0.0742967091364493,
0.868149331745851));
#14885=CARTESIAN_POINT('Ctrl Pts',(-0.54708917182331,-0.115492077056649,
0.85981294420286));
#14886=CARTESIAN_POINT('Ctrl Pts',(-0.560922177770136,-0.141695629206859,
0.850993704737257));
#14887=CARTESIAN_POINT('Ctrl Pts',(-0.590422647829571,-0.181890537957859,
0.830754510485543));
#14888=CARTESIAN_POINT('Ctrl Pts',(-0.609616703125488,-0.201072148666545,
0.816896541396381));
#14889=CARTESIAN_POINT('Ctrl Pts',(-0.641117951819998,-0.223955109275652,
0.792310597819928));
#14890=CARTESIAN_POINT('Ctrl Pts',(-0.657208095763053,-0.232742381310829,
0.779109323683611));
#14891=CARTESIAN_POINT('Ctrl Pts',(-0.68964083160521,-0.244234834628584,
0.750552691816205));
#14892=CARTESIAN_POINT('Ctrl Pts',(-0.705971972091755,-0.246942143572133,
0.735185187071673));
#14893=CARTESIAN_POINT('Ctrl Pts',(-0.735185187071673,-0.246942143572133,
0.705971972091754));
#14894=CARTESIAN_POINT('Ctrl Pts',(-0.750552691816206,-0.244234834628584,
0.689640831605209));
#14895=CARTESIAN_POINT('Ctrl Pts',(-0.779109323683612,-0.232742381310829,
0.657208095763052));
#14896=CARTESIAN_POINT('Ctrl Pts',(-0.792310597819928,-0.223955109275652,
0.641117951819998));
#14897=CARTESIAN_POINT('Ctrl Pts',(-0.816896541396382,-0.201072148666545,
0.609616703125487));
#14898=CARTESIAN_POINT('Ctrl Pts',(-0.830754510485544,-0.181890537957858,
0.590422647829571));
#14899=CARTESIAN_POINT('Ctrl Pts',(-0.850993704737257,-0.141695629206858,
0.560922177770135));
#14900=CARTESIAN_POINT('Ctrl Pts',(-0.859812944202861,-0.115492077056649,
0.547089171823309));
#14901=CARTESIAN_POINT('Ctrl Pts',(-0.868149331745852,-0.0742967091364491,
0.533674141594226));
#14902=CARTESIAN_POINT('Ctrl Pts',(-0.870146645090731,-0.0609922781173483,
0.530395067942936));
#14903=CARTESIAN_POINT('Ctrl Pts',(-0.871530771444223,-0.04763,0.528110872004958));
#14904=CARTESIAN_POINT('',(-0.989696097314,-0.04763,0.242834539687906));
#14905=CARTESIAN_POINT('Origin',(0.,-0.04763,0.));
#14906=CARTESIAN_POINT('',(-1.019052,-0.246942143572133,1.248489836334E-16));
#14907=CARTESIAN_POINT('Ctrl Pts',(-0.989696097314,-0.04763,0.242834539687906));
#14908=CARTESIAN_POINT('Ctrl Pts',(-0.990332542620729,-0.0609922781173483,
0.24024064412003));
#14909=CARTESIAN_POINT('Ctrl Pts',(-0.991238884025248,-0.0742967091364492,
0.236509675094874));
#14910=CARTESIAN_POINT('Ctrl Pts',(-0.994830026707808,-0.115492077056649,
0.221129100087819));
#14911=CARTESIAN_POINT('Ctrl Pts',(-0.998375294985966,-0.141695629206859,
0.205111543747588));
#14912=CARTESIAN_POINT('Ctrl Pts',(-1.00492400591205,-0.181890537957859,
0.169940289819232));
#14913=CARTESIAN_POINT('Ctrl Pts',(-1.00869718865384,-0.201072148666545,
0.1465689792446));
#14914=CARTESIAN_POINT('Ctrl Pts',(-1.01358704779679,-0.223955109275652,
0.106909345252088));
#14915=CARTESIAN_POINT('Ctrl Pts',(-1.0156297872271,-0.232742381310829,
0.0861971848975944));
#14916=CARTESIAN_POINT('Ctrl Pts',(-1.01837060663223,-0.244234834628584,
0.0430711894098825));
#14917=CARTESIAN_POINT('Ctrl Pts',(-1.019052,-0.246942143572133,0.0206568624125608));
#14918=CARTESIAN_POINT('Ctrl Pts',(-1.019052,-0.246942143572133,1.2490009027033E-16));
#14919=CARTESIAN_POINT('',(-1.019052,-0.28578,1.24797876996471E-16));
#14920=CARTESIAN_POINT('',(-1.019052,-0.166705,1.24797876996471E-16));
#14921=CARTESIAN_POINT('Origin',(0.,-0.28578,0.));
#14922=CARTESIAN_POINT('',(-0.989696097314,-0.04763,-0.242834539687906));
#14923=CARTESIAN_POINT('Ctrl Pts',(-1.019052,-0.246942143572133,1.2490009027033E-16));
#14924=CARTESIAN_POINT('Ctrl Pts',(-1.019052,-0.246942143572133,-0.0206568624125605));
#14925=CARTESIAN_POINT('Ctrl Pts',(-1.01837060663223,-0.244234834628584,
-0.0430711894098822));
#14926=CARTESIAN_POINT('Ctrl Pts',(-1.0156297872271,-0.232742381310829,
-0.0861971848975941));
#14927=CARTESIAN_POINT('Ctrl Pts',(-1.01358704779679,-0.223955109275652,
-0.106909345252087));
#14928=CARTESIAN_POINT('Ctrl Pts',(-1.00869718865384,-0.201072148666546,
-0.1465689792446));
#14929=CARTESIAN_POINT('Ctrl Pts',(-1.00492400591205,-0.181890537957859,
-0.169940289819232));
#14930=CARTESIAN_POINT('Ctrl Pts',(-0.998375294985966,-0.141695629206859,
-0.205111543747588));
#14931=CARTESIAN_POINT('Ctrl Pts',(-0.994830026707808,-0.11549207705665,
-0.221129100087819));
#14932=CARTESIAN_POINT('Ctrl Pts',(-0.991238884025248,-0.0742967091364495,
-0.236509675094874));
#14933=CARTESIAN_POINT('Ctrl Pts',(-0.990332542620729,-0.0609922781173484,
-0.24024064412003));
#14934=CARTESIAN_POINT('Ctrl Pts',(-0.989696097314,-0.0476300000000001,
-0.242834539687907));
#14935=CARTESIAN_POINT('',(-0.871530771444223,-0.04763,-0.528110872004958));
#14936=CARTESIAN_POINT('Origin',(0.,-0.04763,0.));
#14937=CARTESIAN_POINT('',(-0.528110872004958,-0.04763,-0.871530771444223));
#14938=CARTESIAN_POINT('Ctrl Pts',(-0.871530771444223,-0.0476300000000001,
-0.528110872004958));
#14939=CARTESIAN_POINT('Ctrl Pts',(-0.87014664509073,-0.0609922781173484,
-0.530395067942936));
#14940=CARTESIAN_POINT('Ctrl Pts',(-0.868149331745851,-0.0742967091364494,
-0.533674141594226));
#14941=CARTESIAN_POINT('Ctrl Pts',(-0.85981294420286,-0.115492077056649,
-0.54708917182331));
#14942=CARTESIAN_POINT('Ctrl Pts',(-0.850993704737257,-0.141695629206859,
-0.560922177770136));
#14943=CARTESIAN_POINT('Ctrl Pts',(-0.830754510485543,-0.181890537957859,
-0.590422647829571));
#14944=CARTESIAN_POINT('Ctrl Pts',(-0.816896541396381,-0.201072148666546,
-0.609616703125488));
#14945=CARTESIAN_POINT('Ctrl Pts',(-0.792310597819928,-0.223955109275652,
-0.641117951819999));
#14946=CARTESIAN_POINT('Ctrl Pts',(-0.779109323683611,-0.232742381310829,
-0.657208095763053));
#14947=CARTESIAN_POINT('Ctrl Pts',(-0.750552691816205,-0.244234834628584,
-0.68964083160521));
#14948=CARTESIAN_POINT('Ctrl Pts',(-0.735185187071673,-0.246942143572133,
-0.705971972091755));
#14949=CARTESIAN_POINT('Ctrl Pts',(-0.705971972091754,-0.246942143572133,
-0.735185187071673));
#14950=CARTESIAN_POINT('Ctrl Pts',(-0.68964083160521,-0.244234834628584,
-0.750552691816206));
#14951=CARTESIAN_POINT('Ctrl Pts',(-0.657208095763052,-0.232742381310829,
-0.779109323683612));
#14952=CARTESIAN_POINT('Ctrl Pts',(-0.641117951819998,-0.223955109275652,
-0.792310597819928));
#14953=CARTESIAN_POINT('Ctrl Pts',(-0.609616703125488,-0.201072148666545,
-0.816896541396381));
#14954=CARTESIAN_POINT('Ctrl Pts',(-0.590422647829571,-0.181890537957859,
-0.830754510485543));
#14955=CARTESIAN_POINT('Ctrl Pts',(-0.560922177770136,-0.141695629206859,
-0.850993704737257));
#14956=CARTESIAN_POINT('Ctrl Pts',(-0.54708917182331,-0.115492077056649,
-0.85981294420286));
#14957=CARTESIAN_POINT('Ctrl Pts',(-0.533674141594226,-0.0742967091364494,
-0.868149331745852));
#14958=CARTESIAN_POINT('Ctrl Pts',(-0.530395067942936,-0.0609922781173484,
-0.870146645090731));
#14959=CARTESIAN_POINT('Ctrl Pts',(-0.528110872004958,-0.0476300000000001,
-0.871530771444223));
#14960=CARTESIAN_POINT('',(-0.242834539687906,-0.04763,-0.989696097314));
#14961=CARTESIAN_POINT('Origin',(0.,-0.04763,0.));
#14962=CARTESIAN_POINT('',(0.242834539687906,-0.04763,-0.989696097314));
#14963=CARTESIAN_POINT('Ctrl Pts',(-0.242834539687907,-0.04763,-0.989696097314));
#14964=CARTESIAN_POINT('Ctrl Pts',(-0.24024064412003,-0.0609922781173483,
-0.990332542620729));
#14965=CARTESIAN_POINT('Ctrl Pts',(-0.236509675094874,-0.0742967091364493,
-0.991238884025248));
#14966=CARTESIAN_POINT('Ctrl Pts',(-0.221129100087819,-0.115492077056649,
-0.994830026707808));
#14967=CARTESIAN_POINT('Ctrl Pts',(-0.205111543747588,-0.141695629206859,
-0.998375294985966));
#14968=CARTESIAN_POINT('Ctrl Pts',(-0.169940289819232,-0.181890537957859,
-1.00492400591205));
#14969=CARTESIAN_POINT('Ctrl Pts',(-0.1465689792446,-0.201072148666545,
-1.00869718865384));
#14970=CARTESIAN_POINT('Ctrl Pts',(-0.106909345252087,-0.223955109275652,
-1.01358704779679));
#14971=CARTESIAN_POINT('Ctrl Pts',(-0.0861971848975942,-0.232742381310829,
-1.0156297872271));
#14972=CARTESIAN_POINT('Ctrl Pts',(-0.0430711894098823,-0.244234834628584,
-1.01837060663223));
#14973=CARTESIAN_POINT('Ctrl Pts',(-0.0206568624125606,-0.246942143572133,
-1.019052));
#14974=CARTESIAN_POINT('Ctrl Pts',(0.0206568624125607,-0.246942143572133,
-1.019052));
#14975=CARTESIAN_POINT('Ctrl Pts',(0.0430711894098824,-0.244234834628584,
-1.01837060663223));
#14976=CARTESIAN_POINT('Ctrl Pts',(0.0861971848975943,-0.232742381310829,
-1.0156297872271));
#14977=CARTESIAN_POINT('Ctrl Pts',(0.106909345252088,-0.223955109275652,
-1.01358704779679));
#14978=CARTESIAN_POINT('Ctrl Pts',(0.1465689792446,-0.201072148666545,-1.00869718865384));
#14979=CARTESIAN_POINT('Ctrl Pts',(0.169940289819232,-0.181890537957859,
-1.00492400591205));
#14980=CARTESIAN_POINT('Ctrl Pts',(0.205111543747588,-0.141695629206859,
-0.998375294985966));
#14981=CARTESIAN_POINT('Ctrl Pts',(0.221129100087819,-0.115492077056649,
-0.994830026707808));
#14982=CARTESIAN_POINT('Ctrl Pts',(0.236509675094874,-0.0742967091364493,
-0.991238884025248));
#14983=CARTESIAN_POINT('Ctrl Pts',(0.24024064412003,-0.0609922781173484,
-0.990332542620729));
#14984=CARTESIAN_POINT('Ctrl Pts',(0.242834539687907,-0.04763,-0.989696097314));
#14985=CARTESIAN_POINT('',(0.528110872004958,-0.04763,-0.871530771444223));
#14986=CARTESIAN_POINT('Origin',(0.,-0.04763,0.));
#14987=CARTESIAN_POINT('',(0.871530771444223,-0.04763,-0.528110872004958));
#14988=CARTESIAN_POINT('Ctrl Pts',(0.528110872004958,-0.0476300000000001,
-0.871530771444223));
#14989=CARTESIAN_POINT('Ctrl Pts',(0.530395067942936,-0.0609922781173484,
-0.870146645090731));
#14990=CARTESIAN_POINT('Ctrl Pts',(0.533674141594226,-0.0742967091364493,
-0.868149331745851));
#14991=CARTESIAN_POINT('Ctrl Pts',(0.54708917182331,-0.115492077056649,
-0.85981294420286));
#14992=CARTESIAN_POINT('Ctrl Pts',(0.560922177770136,-0.141695629206859,
-0.850993704737257));
#14993=CARTESIAN_POINT('Ctrl Pts',(0.590422647829571,-0.181890537957859,
-0.830754510485543));
#14994=CARTESIAN_POINT('Ctrl Pts',(0.609616703125488,-0.201072148666545,
-0.816896541396381));
#14995=CARTESIAN_POINT('Ctrl Pts',(0.641117951819998,-0.223955109275652,
-0.792310597819928));
#14996=CARTESIAN_POINT('Ctrl Pts',(0.657208095763053,-0.232742381310829,
-0.779109323683612));
#14997=CARTESIAN_POINT('Ctrl Pts',(0.68964083160521,-0.244234834628584,
-0.750552691816206));
#14998=CARTESIAN_POINT('Ctrl Pts',(0.705971972091755,-0.246942143572133,
-0.735185187071673));
#14999=CARTESIAN_POINT('Ctrl Pts',(0.735185187071673,-0.246942143572133,
-0.705971972091754));
#15000=CARTESIAN_POINT('Ctrl Pts',(0.750552691816206,-0.244234834628584,
-0.68964083160521));
#15001=CARTESIAN_POINT('Ctrl Pts',(0.779109323683612,-0.232742381310829,
-0.657208095763053));
#15002=CARTESIAN_POINT('Ctrl Pts',(0.792310597819928,-0.223955109275652,
-0.641117951819998));
#15003=CARTESIAN_POINT('Ctrl Pts',(0.816896541396381,-0.201072148666545,
-0.609616703125488));
#15004=CARTESIAN_POINT('Ctrl Pts',(0.830754510485543,-0.181890537957859,
-0.590422647829571));
#15005=CARTESIAN_POINT('Ctrl Pts',(0.850993704737257,-0.141695629206859,
-0.560922177770136));
#15006=CARTESIAN_POINT('Ctrl Pts',(0.85981294420286,-0.115492077056649,
-0.54708917182331));
#15007=CARTESIAN_POINT('Ctrl Pts',(0.868149331745851,-0.0742967091364493,
-0.533674141594226));
#15008=CARTESIAN_POINT('Ctrl Pts',(0.870146645090731,-0.0609922781173484,
-0.530395067942936));
#15009=CARTESIAN_POINT('Ctrl Pts',(0.871530771444223,-0.0476300000000001,
-0.528110872004958));
#15010=CARTESIAN_POINT('',(0.989696097314,-0.04763,-0.242834539687906));
#15011=CARTESIAN_POINT('Origin',(0.,-0.04763,0.));
#15012=CARTESIAN_POINT('',(0.989696097314,-0.04763,0.242834539687906));
#15013=CARTESIAN_POINT('Ctrl Pts',(0.989696097314,-0.04763,-0.242834539687907));
#15014=CARTESIAN_POINT('Ctrl Pts',(0.990332542620729,-0.0609922781173483,
-0.24024064412003));
#15015=CARTESIAN_POINT('Ctrl Pts',(0.991238884025248,-0.0742967091364493,
-0.236509675094874));
#15016=CARTESIAN_POINT('Ctrl Pts',(0.994830026707808,-0.115492077056649,
-0.221129100087819));
#15017=CARTESIAN_POINT('Ctrl Pts',(0.998375294985966,-0.141695629206859,
-0.205111543747588));
#15018=CARTESIAN_POINT('Ctrl Pts',(1.00492400591205,-0.181890537957859,
-0.169940289819232));
#15019=CARTESIAN_POINT('Ctrl Pts',(1.00869718865384,-0.201072148666545,
-0.1465689792446));
#15020=CARTESIAN_POINT('Ctrl Pts',(1.01358704779679,-0.223955109275652,
-0.106909345252087));
#15021=CARTESIAN_POINT('Ctrl Pts',(1.0156297872271,-0.232742381310829,-0.0861971848975942));
#15022=CARTESIAN_POINT('Ctrl Pts',(1.01837060663223,-0.244234834628584,
-0.0430711894098823));
#15023=CARTESIAN_POINT('Ctrl Pts',(1.019052,-0.246942143572133,-0.0206568624125607));
#15024=CARTESIAN_POINT('Ctrl Pts',(1.019052,-0.246942143572133,0.0206568624125607));
#15025=CARTESIAN_POINT('Ctrl Pts',(1.01837060663223,-0.244234834628584,
0.0430711894098823));
#15026=CARTESIAN_POINT('Ctrl Pts',(1.0156297872271,-0.232742381310829,0.0861971848975942));
#15027=CARTESIAN_POINT('Ctrl Pts',(1.01358704779679,-0.223955109275652,
0.106909345252087));
#15028=CARTESIAN_POINT('Ctrl Pts',(1.00869718865384,-0.201072148666545,
0.1465689792446));
#15029=CARTESIAN_POINT('Ctrl Pts',(1.00492400591205,-0.181890537957859,
0.169940289819232));
#15030=CARTESIAN_POINT('Ctrl Pts',(0.998375294985966,-0.141695629206859,
0.205111543747588));
#15031=CARTESIAN_POINT('Ctrl Pts',(0.994830026707808,-0.115492077056649,
0.221129100087819));
#15032=CARTESIAN_POINT('Ctrl Pts',(0.991238884025248,-0.0742967091364492,
0.236509675094874));
#15033=CARTESIAN_POINT('Ctrl Pts',(0.990332542620729,-0.0609922781173483,
0.24024064412003));
#15034=CARTESIAN_POINT('Ctrl Pts',(0.989696097314,-0.04763,0.242834539687907));
#15035=CARTESIAN_POINT('Origin',(0.,-0.04763,0.));
#15036=CARTESIAN_POINT('Origin',(0.,-0.04763,0.));
#15037=CARTESIAN_POINT('',(0.238183666596899,-0.04763,0.951592097314));
#15038=CARTESIAN_POINT('Origin',(0.,-0.04763,0.));
#15039=CARTESIAN_POINT('Origin',(-1.94289029309402E-16,-0.04763,1.));
#15040=CARTESIAN_POINT('Origin',(-1.94289029309402E-16,0.,1.));
#15041=CARTESIAN_POINT('',(-0.2381836665969,-0.04763,0.951592097314));
#15042=CARTESIAN_POINT('Ctrl Pts',(-0.238183666596899,-0.0476299999999999,
0.951592097314));
#15043=CARTESIAN_POINT('Ctrl Pts',(-0.233157223576062,-0.0740444353928835,
0.952850216871763));
#15044=CARTESIAN_POINT('Ctrl Pts',(-0.223801617934946,-0.0999305678883309,
0.955173119738174));
#15045=CARTESIAN_POINT('Ctrl Pts',(-0.199966927975188,-0.142345102874864,
0.960411259488514));
#15046=CARTESIAN_POINT('Ctrl Pts',(-0.1868781821531,-0.159766064500479,
0.963103647174702));
#15047=CARTESIAN_POINT('Ctrl Pts',(-0.15681442133453,-0.190326085855194,
0.968453058988463));
#15048=CARTESIAN_POINT('Ctrl Pts',(-0.139836317888043,-0.203463743702801,
0.971100730005489));
#15049=CARTESIAN_POINT('Ctrl Pts',(-0.104422493053067,-0.224161999508995,
0.975530745318961));
#15050=CARTESIAN_POINT('Ctrl Pts',(-0.0842175114474176,-0.232861760990032,
0.977553872336861));
#15051=CARTESIAN_POINT('Ctrl Pts',(-0.0421062857595701,-0.244251601209411,
0.980270995488453));
#15052=CARTESIAN_POINT('Ctrl Pts',(-0.0201990724523197,-0.246942143572133,
0.980948));
#15053=CARTESIAN_POINT('Ctrl Pts',(0.020199072452319,-0.246942143572133,
0.980948));
#15054=CARTESIAN_POINT('Ctrl Pts',(0.0421062857595694,-0.244251601209411,
0.980270995488454));
#15055=CARTESIAN_POINT('Ctrl Pts',(0.0842175114474169,-0.232861760990032,
0.977553872336861));
#15056=CARTESIAN_POINT('Ctrl Pts',(0.104422493053067,-0.224161999508995,
0.975530745318961));
#15057=CARTESIAN_POINT('Ctrl Pts',(0.139836317888042,-0.203463743702801,
0.971100730005489));
#15058=CARTESIAN_POINT('Ctrl Pts',(0.15681442133453,-0.190326085855194,
0.968453058988463));
#15059=CARTESIAN_POINT('Ctrl Pts',(0.1868781821531,-0.15976606450048,0.963103647174702));
#15060=CARTESIAN_POINT('Ctrl Pts',(0.199966927975188,-0.142345102874864,
0.960411259488514));
#15061=CARTESIAN_POINT('Ctrl Pts',(0.223801617934945,-0.0999305678883309,
0.955173119738174));
#15062=CARTESIAN_POINT('Ctrl Pts',(0.233157223576061,-0.0740444353928835,
0.952850216871763));
#15063=CARTESIAN_POINT('Ctrl Pts',(0.238183666596899,-0.0476299999999999,
0.951592097314));
#15064=CARTESIAN_POINT('Origin',(-1.94289029309402E-16,-0.04763,1.));
#15065=CARTESIAN_POINT('Origin',(0.,-0.04763,0.));
#15066=CARTESIAN_POINT('',(-0.504455939115715,-0.04763,0.841298510752802));
#15067=CARTESIAN_POINT('Origin',(0.,-0.04763,0.));
#15068=CARTESIAN_POINT('Origin',(-0.707106781186548,-0.04763,0.707106781186547));
#15069=CARTESIAN_POINT('Origin',(-0.707106781186548,0.,0.707106781186547));
#15070=CARTESIAN_POINT('',(-0.841298510752802,-0.04763,0.504455939115715));
#15071=CARTESIAN_POINT('Ctrl Pts',(-0.841298510752802,-0.04763,0.504455939115715));
#15072=CARTESIAN_POINT('Ctrl Pts',(-0.838633903678357,-0.0740444353928835,
0.508899795931835));
#15073=CARTESIAN_POINT('Ctrl Pts',(-0.833661031856294,-0.0999305678883309,
0.517157748491652));
#15074=CARTESIAN_POINT('Ctrl Pts',(-0.820511285096538,-0.142345102874864,
0.537715343527944));
#15075=CARTESIAN_POINT('Ctrl Pts',(-0.813159949759,-0.159766064500479,0.548874290046456));
#15076=CARTESIAN_POINT('Ctrl Pts',(-0.795684265985089,-0.190326085855194,
0.573915184558107));
#15077=CARTESIAN_POINT('Ctrl Pts',(-0.78555112003688,-0.203463743702801,
0.587792702767295));
#15078=CARTESIAN_POINT('Ctrl Pts',(-0.763642258217233,-0.224161999508995,
0.615966552324775));
#15079=CARTESIAN_POINT('Ctrl Pts',(-0.750785745543687,-0.232861760990032,
0.631684198665438));
#15080=CARTESIAN_POINT('Ctrl Pts',(-0.722929908501543,-0.244251601209411,
0.663382628119203));
#15081=CARTESIAN_POINT('Ctrl Pts',(-0.707917883896095,-0.246942143572133,
0.679352081686668));
#15082=CARTESIAN_POINT('Ctrl Pts',(-0.679352081686668,-0.246942143572133,
0.707917883896095));
#15083=CARTESIAN_POINT('Ctrl Pts',(-0.663382628119203,-0.244251601209411,
0.722929908501544));
#15084=CARTESIAN_POINT('Ctrl Pts',(-0.631684198665438,-0.232861760990031,
0.750785745543687));
#15085=CARTESIAN_POINT('Ctrl Pts',(-0.615966552324775,-0.224161999508995,
0.763642258217233));
#15086=CARTESIAN_POINT('Ctrl Pts',(-0.587792702767295,-0.203463743702801,
0.78555112003688));
#15087=CARTESIAN_POINT('Ctrl Pts',(-0.573915184558107,-0.190326085855194,
0.795684265985088));
#15088=CARTESIAN_POINT('Ctrl Pts',(-0.548874290046456,-0.159766064500479,
0.813159949759));
#15089=CARTESIAN_POINT('Ctrl Pts',(-0.537715343527944,-0.142345102874864,
0.820511285096538));
#15090=CARTESIAN_POINT('Ctrl Pts',(-0.517157748491652,-0.0999305678883309,
0.833661031856294));
#15091=CARTESIAN_POINT('Ctrl Pts',(-0.508899795931835,-0.0740444353928835,
0.838633903678357));
#15092=CARTESIAN_POINT('Ctrl Pts',(-0.504455939115716,-0.04763,0.841298510752801));
#15093=CARTESIAN_POINT('Origin',(-0.707106781186548,-0.04763,0.707106781186547));
#15094=CARTESIAN_POINT('Origin',(0.,-0.04763,0.));
#15095=CARTESIAN_POINT('',(-0.951592097314,-0.04763,0.238183666596899));
#15096=CARTESIAN_POINT('Origin',(0.,-0.04763,0.));
#15097=CARTESIAN_POINT('Origin',(-1.,-0.04763,-1.11022302462516E-16));
#15098=CARTESIAN_POINT('Origin',(-1.,0.,-1.11022302462516E-16));
#15099=CARTESIAN_POINT('',(-0.951592097314,-0.04763,-0.2381836665969));
#15100=CARTESIAN_POINT('',(-0.980948,-0.246942143572133,1.08514323328844E-18));
#15101=CARTESIAN_POINT('Ctrl Pts',(-0.951592097314,-0.04763,-0.238183666596899));
#15102=CARTESIAN_POINT('Ctrl Pts',(-0.952850216871763,-0.0740444353928835,
-0.233157223576062));
#15103=CARTESIAN_POINT('Ctrl Pts',(-0.955173119738174,-0.0999305678883309,
-0.223801617934946));
#15104=CARTESIAN_POINT('Ctrl Pts',(-0.960411259488514,-0.142345102874864,
-0.199966927975188));
#15105=CARTESIAN_POINT('Ctrl Pts',(-0.963103647174702,-0.159766064500479,
-0.1868781821531));
#15106=CARTESIAN_POINT('Ctrl Pts',(-0.968453058988463,-0.190326085855194,
-0.15681442133453));
#15107=CARTESIAN_POINT('Ctrl Pts',(-0.971100730005489,-0.203463743702801,
-0.139836317888043));
#15108=CARTESIAN_POINT('Ctrl Pts',(-0.975530745318961,-0.224161999508995,
-0.104422493053067));
#15109=CARTESIAN_POINT('Ctrl Pts',(-0.977553872336861,-0.232861760990032,
-0.0842175114474175));
#15110=CARTESIAN_POINT('Ctrl Pts',(-0.980270995488453,-0.244251601209411,
-0.0421062857595699));
#15111=CARTESIAN_POINT('Ctrl Pts',(-0.980948,-0.246942143572133,-0.0201990724523195));
#15112=CARTESIAN_POINT('Ctrl Pts',(-0.980948,-0.246942143572133,-1.17961196366423E-16));
#15113=CARTESIAN_POINT('Origin',(-1.,-0.04763,-1.11022302462516E-16));
#15114=CARTESIAN_POINT('Ctrl Pts',(-0.980948,-0.246942143572133,-1.17961196366423E-16));
#15115=CARTESIAN_POINT('Ctrl Pts',(-0.980948,-0.246942143572133,0.0201990724523192));
#15116=CARTESIAN_POINT('Ctrl Pts',(-0.980270995488453,-0.244251601209411,
0.0421062857595695));
#15117=CARTESIAN_POINT('Ctrl Pts',(-0.977553872336861,-0.232861760990032,
0.0842175114474169));
#15118=CARTESIAN_POINT('Ctrl Pts',(-0.975530745318961,-0.224161999508995,
0.104422493053066));
#15119=CARTESIAN_POINT('Ctrl Pts',(-0.971100730005489,-0.203463743702801,
0.139836317888042));
#15120=CARTESIAN_POINT('Ctrl Pts',(-0.968453058988463,-0.190326085855194,
0.15681442133453));
#15121=CARTESIAN_POINT('Ctrl Pts',(-0.963103647174702,-0.15976606450048,
0.1868781821531));
#15122=CARTESIAN_POINT('Ctrl Pts',(-0.960411259488514,-0.142345102874864,
0.199966927975188));
#15123=CARTESIAN_POINT('Ctrl Pts',(-0.955173119738174,-0.099930567888331,
0.223801617934945));
#15124=CARTESIAN_POINT('Ctrl Pts',(-0.952850216871763,-0.0740444353928835,
0.233157223576061));
#15125=CARTESIAN_POINT('Ctrl Pts',(-0.951592097314,-0.04763,0.238183666596899));
#15126=CARTESIAN_POINT('Origin',(0.,-0.04763,0.));
#15127=CARTESIAN_POINT('',(-0.841298510752802,-0.04763,-0.504455939115715));
#15128=CARTESIAN_POINT('Origin',(0.,-0.04763,0.));
#15129=CARTESIAN_POINT('Origin',(-0.707106781186547,-0.04763,-0.707106781186548));
#15130=CARTESIAN_POINT('Origin',(-0.707106781186547,0.,-0.707106781186548));
#15131=CARTESIAN_POINT('',(-0.504455939115715,-0.04763,-0.841298510752802));
#15132=CARTESIAN_POINT('Ctrl Pts',(-0.504455939115715,-0.04763,-0.841298510752802));
#15133=CARTESIAN_POINT('Ctrl Pts',(-0.508899795931835,-0.0740444353928835,
-0.838633903678357));
#15134=CARTESIAN_POINT('Ctrl Pts',(-0.517157748491652,-0.0999305678883309,
-0.833661031856294));
#15135=CARTESIAN_POINT('Ctrl Pts',(-0.537715343527944,-0.142345102874864,
-0.820511285096538));
#15136=CARTESIAN_POINT('Ctrl Pts',(-0.548874290046456,-0.159766064500479,
-0.813159949759));
#15137=CARTESIAN_POINT('Ctrl Pts',(-0.573915184558107,-0.190326085855194,
-0.795684265985089));
#15138=CARTESIAN_POINT('Ctrl Pts',(-0.587792702767295,-0.203463743702801,
-0.78555112003688));
#15139=CARTESIAN_POINT('Ctrl Pts',(-0.615966552324775,-0.224161999508995,
-0.763642258217233));
#15140=CARTESIAN_POINT('Ctrl Pts',(-0.631684198665438,-0.232861760990032,
-0.750785745543687));
#15141=CARTESIAN_POINT('Ctrl Pts',(-0.663382628119203,-0.244251601209411,
-0.722929908501543));
#15142=CARTESIAN_POINT('Ctrl Pts',(-0.679352081686668,-0.246942143572133,
-0.707917883896095));
#15143=CARTESIAN_POINT('Ctrl Pts',(-0.707917883896095,-0.246942143572133,
-0.679352081686668));
#15144=CARTESIAN_POINT('Ctrl Pts',(-0.722929908501543,-0.244251601209411,
-0.663382628119203));
#15145=CARTESIAN_POINT('Ctrl Pts',(-0.750785745543687,-0.232861760990032,
-0.631684198665439));
#15146=CARTESIAN_POINT('Ctrl Pts',(-0.763642258217232,-0.224161999508995,
-0.615966552324775));
#15147=CARTESIAN_POINT('Ctrl Pts',(-0.78555112003688,-0.203463743702801,
-0.587792702767295));
#15148=CARTESIAN_POINT('Ctrl Pts',(-0.795684265985088,-0.190326085855194,
-0.573915184558107));
#15149=CARTESIAN_POINT('Ctrl Pts',(-0.813159949759,-0.15976606450048,-0.548874290046456));
#15150=CARTESIAN_POINT('Ctrl Pts',(-0.820511285096538,-0.142345102874864,
-0.537715343527944));
#15151=CARTESIAN_POINT('Ctrl Pts',(-0.833661031856294,-0.0999305678883311,
-0.517157748491652));
#15152=CARTESIAN_POINT('Ctrl Pts',(-0.838633903678357,-0.0740444353928836,
-0.508899795931835));
#15153=CARTESIAN_POINT('Ctrl Pts',(-0.841298510752801,-0.04763,-0.504455939115715));
#15154=CARTESIAN_POINT('Origin',(-0.707106781186547,-0.04763,-0.707106781186548));
#15155=CARTESIAN_POINT('Origin',(0.,-0.04763,0.));
#15156=CARTESIAN_POINT('',(-0.238183666596899,-0.04763,-0.951592097314));
#15157=CARTESIAN_POINT('Origin',(0.,-0.04763,0.));
#15158=CARTESIAN_POINT('Origin',(5.55111512312578E-17,-0.04763,-1.));
#15159=CARTESIAN_POINT('Origin',(5.55111512312578E-17,0.,-1.));
#15160=CARTESIAN_POINT('',(0.238183666596899,-0.04763,-0.951592097314));
#15161=CARTESIAN_POINT('Ctrl Pts',(0.238183666596899,-0.04763,-0.951592097314));
#15162=CARTESIAN_POINT('Ctrl Pts',(0.233157223576062,-0.0740444353928835,
-0.952850216871763));
#15163=CARTESIAN_POINT('Ctrl Pts',(0.223801617934946,-0.099930567888331,
-0.955173119738174));
#15164=CARTESIAN_POINT('Ctrl Pts',(0.199966927975188,-0.142345102874864,
-0.960411259488514));
#15165=CARTESIAN_POINT('Ctrl Pts',(0.1868781821531,-0.15976606450048,-0.963103647174702));
#15166=CARTESIAN_POINT('Ctrl Pts',(0.15681442133453,-0.190326085855194,
-0.968453058988463));
#15167=CARTESIAN_POINT('Ctrl Pts',(0.139836317888042,-0.203463743702801,
-0.971100730005489));
#15168=CARTESIAN_POINT('Ctrl Pts',(0.104422493053067,-0.224161999508995,
-0.975530745318961));
#15169=CARTESIAN_POINT('Ctrl Pts',(0.0842175114474173,-0.232861760990032,
-0.977553872336861));
#15170=CARTESIAN_POINT('Ctrl Pts',(0.0421062857595698,-0.244251601209411,
-0.980270995488453));
#15171=CARTESIAN_POINT('Ctrl Pts',(0.0201990724523194,-0.246942143572133,
-0.980948));
#15172=CARTESIAN_POINT('Ctrl Pts',(-0.0201990724523193,-0.246942143572133,
-0.980948));
#15173=CARTESIAN_POINT('Ctrl Pts',(-0.0421062857595697,-0.244251601209411,
-0.980270995488453));
#15174=CARTESIAN_POINT('Ctrl Pts',(-0.0842175114474171,-0.232861760990032,
-0.977553872336861));
#15175=CARTESIAN_POINT('Ctrl Pts',(-0.104422493053067,-0.224161999508995,
-0.975530745318961));
#15176=CARTESIAN_POINT('Ctrl Pts',(-0.139836317888042,-0.203463743702801,
-0.971100730005489));
#15177=CARTESIAN_POINT('Ctrl Pts',(-0.15681442133453,-0.190326085855194,
-0.968453058988463));
#15178=CARTESIAN_POINT('Ctrl Pts',(-0.1868781821531,-0.15976606450048,-0.963103647174702));
#15179=CARTESIAN_POINT('Ctrl Pts',(-0.199966927975188,-0.142345102874864,
-0.960411259488514));
#15180=CARTESIAN_POINT('Ctrl Pts',(-0.223801617934945,-0.099930567888331,
-0.955173119738174));
#15181=CARTESIAN_POINT('Ctrl Pts',(-0.233157223576062,-0.0740444353928835,
-0.952850216871763));
#15182=CARTESIAN_POINT('Ctrl Pts',(-0.238183666596899,-0.0476299999999999,
-0.951592097314));
#15183=CARTESIAN_POINT('Origin',(5.55111512312578E-17,-0.04763,-1.));
#15184=CARTESIAN_POINT('Origin',(0.,-0.04763,0.));
#15185=CARTESIAN_POINT('',(0.504455939115715,-0.04763,-0.841298510752802));
#15186=CARTESIAN_POINT('Origin',(0.,-0.04763,0.));
#15187=CARTESIAN_POINT('Origin',(0.707106781186548,-0.04763,-0.707106781186547));
#15188=CARTESIAN_POINT('Origin',(0.707106781186548,0.,-0.707106781186547));
#15189=CARTESIAN_POINT('',(0.841298510752802,-0.04763,-0.504455939115715));
#15190=CARTESIAN_POINT('Ctrl Pts',(0.841298510752802,-0.04763,-0.504455939115715));
#15191=CARTESIAN_POINT('Ctrl Pts',(0.838633903678357,-0.0740444353928835,
-0.508899795931835));
#15192=CARTESIAN_POINT('Ctrl Pts',(0.833661031856294,-0.0999305678883309,
-0.517157748491652));
#15193=CARTESIAN_POINT('Ctrl Pts',(0.820511285096538,-0.142345102874864,
-0.537715343527944));
#15194=CARTESIAN_POINT('Ctrl Pts',(0.813159949759,-0.159766064500479,-0.548874290046456));
#15195=CARTESIAN_POINT('Ctrl Pts',(0.795684265985088,-0.190326085855194,
-0.573915184558107));
#15196=CARTESIAN_POINT('Ctrl Pts',(0.78555112003688,-0.203463743702801,
-0.587792702767295));
#15197=CARTESIAN_POINT('Ctrl Pts',(0.763642258217233,-0.224161999508995,
-0.615966552324775));
#15198=CARTESIAN_POINT('Ctrl Pts',(0.750785745543687,-0.232861760990032,
-0.631684198665438));
#15199=CARTESIAN_POINT('Ctrl Pts',(0.722929908501543,-0.244251601209411,
-0.663382628119203));
#15200=CARTESIAN_POINT('Ctrl Pts',(0.707917883896095,-0.246942143572133,
-0.679352081686668));
#15201=CARTESIAN_POINT('Ctrl Pts',(0.679352081686668,-0.246942143572133,
-0.707917883896095));
#15202=CARTESIAN_POINT('Ctrl Pts',(0.663382628119203,-0.244251601209411,
-0.722929908501543));
#15203=CARTESIAN_POINT('Ctrl Pts',(0.631684198665438,-0.232861760990032,
-0.750785745543687));
#15204=CARTESIAN_POINT('Ctrl Pts',(0.615966552324775,-0.224161999508995,
-0.763642258217232));
#15205=CARTESIAN_POINT('Ctrl Pts',(0.587792702767295,-0.203463743702801,
-0.78555112003688));
#15206=CARTESIAN_POINT('Ctrl Pts',(0.573915184558107,-0.190326085855194,
-0.795684265985088));
#15207=CARTESIAN_POINT('Ctrl Pts',(0.548874290046456,-0.159766064500479,
-0.813159949759));
#15208=CARTESIAN_POINT('Ctrl Pts',(0.537715343527944,-0.142345102874864,
-0.820511285096538));
#15209=CARTESIAN_POINT('Ctrl Pts',(0.517157748491652,-0.099930567888331,
-0.833661031856294));
#15210=CARTESIAN_POINT('Ctrl Pts',(0.508899795931835,-0.0740444353928835,
-0.838633903678357));
#15211=CARTESIAN_POINT('Ctrl Pts',(0.504455939115715,-0.04763,-0.841298510752801));
#15212=CARTESIAN_POINT('Origin',(0.707106781186548,-0.04763,-0.707106781186547));
#15213=CARTESIAN_POINT('Origin',(0.,-0.166705,0.));
#15214=CARTESIAN_POINT('',(-0.980948,-0.28578,1.20131482833E-16));
#15215=CARTESIAN_POINT('Origin',(0.,-0.28578,0.));
#15216=CARTESIAN_POINT('',(-0.980948,-0.166705,1.20131482833E-16));
#15217=CARTESIAN_POINT('',(0.951592097314,-0.04763,0.238183666596899));
#15218=CARTESIAN_POINT('Origin',(0.,-0.04763,0.));
#15219=CARTESIAN_POINT('',(0.951592097314,-0.04763,-0.238183666596899));
#15220=CARTESIAN_POINT('Ctrl Pts',(0.951592097314,-0.04763,0.238183666596899));
#15221=CARTESIAN_POINT('Ctrl Pts',(0.952850216871763,-0.0740444353928835,
0.233157223576062));
#15222=CARTESIAN_POINT('Ctrl Pts',(0.955173119738174,-0.099930567888331,
0.223801617934945));
#15223=CARTESIAN_POINT('Ctrl Pts',(0.960411259488514,-0.142345102874864,
0.199966927975188));
#15224=CARTESIAN_POINT('Ctrl Pts',(0.963103647174702,-0.15976606450048,
0.1868781821531));
#15225=CARTESIAN_POINT('Ctrl Pts',(0.968453058988463,-0.190326085855194,
0.15681442133453));
#15226=CARTESIAN_POINT('Ctrl Pts',(0.971100730005489,-0.203463743702801,
0.139836317888042));
#15227=CARTESIAN_POINT('Ctrl Pts',(0.975530745318961,-0.224161999508995,
0.104422493053067));
#15228=CARTESIAN_POINT('Ctrl Pts',(0.977553872336861,-0.232861760990032,
0.0842175114474172));
#15229=CARTESIAN_POINT('Ctrl Pts',(0.980270995488453,-0.244251601209411,
0.0421062857595697));
#15230=CARTESIAN_POINT('Ctrl Pts',(0.980948,-0.246942143572133,0.0201990724523194));
#15231=CARTESIAN_POINT('Ctrl Pts',(0.980948,-0.246942143572133,-0.0201990724523194));
#15232=CARTESIAN_POINT('Ctrl Pts',(0.980270995488453,-0.244251601209411,
-0.0421062857595697));
#15233=CARTESIAN_POINT('Ctrl Pts',(0.977553872336861,-0.232861760990032,
-0.0842175114474172));
#15234=CARTESIAN_POINT('Ctrl Pts',(0.975530745318961,-0.224161999508995,
-0.104422493053067));
#15235=CARTESIAN_POINT('Ctrl Pts',(0.971100730005489,-0.203463743702801,
-0.139836317888042));
#15236=CARTESIAN_POINT('Ctrl Pts',(0.968453058988463,-0.190326085855194,
-0.15681442133453));
#15237=CARTESIAN_POINT('Ctrl Pts',(0.963103647174702,-0.15976606450048,
-0.1868781821531));
#15238=CARTESIAN_POINT('Ctrl Pts',(0.960411259488514,-0.142345102874864,
-0.199966927975188));
#15239=CARTESIAN_POINT('Ctrl Pts',(0.955173119738174,-0.099930567888331,
-0.223801617934945));
#15240=CARTESIAN_POINT('Ctrl Pts',(0.952850216871763,-0.0740444353928835,
-0.233157223576062));
#15241=CARTESIAN_POINT('Ctrl Pts',(0.951592097314,-0.0476299999999999,-0.238183666596899));
#15242=CARTESIAN_POINT('Origin',(0.,-0.04763,0.));
#15243=CARTESIAN_POINT('Origin',(0.,-0.04763,0.));
#15244=CARTESIAN_POINT('Origin',(1.,-0.04763,0.));
#15245=CARTESIAN_POINT('Origin',(1.,0.,0.));
#15246=CARTESIAN_POINT('Origin',(1.,-0.04763,0.));
#15247=CARTESIAN_POINT('Origin',(0.,-0.28578,0.));
#15248=CARTESIAN_POINT('Origin',(0.,-0.04763,0.));
#17753=UNCERTAINTY_MEASURE_WITH_UNIT(LENGTH_MEASURE(0.001),#17831,
'DISTANCE_ACCURACY_VALUE',
'Maximum model space distance between geometric entities at asserted c
onnectivities');
#17780=UNCERTAINTY_MEASURE_WITH_UNIT(LENGTH_MEASURE(0.001),#17831,
'DISTANCE_ACCURACY_VALUE',
'Maximum model space distance between geometric entities at asserted c
onnectivities');
#17803=(
GEOMETRIC_REPRESENTATION_CONTEXT(3)
GLOBAL_UNCERTAINTY_ASSIGNED_CONTEXT((#17753))
GLOBAL_UNIT_ASSIGNED_CONTEXT((#17831,#17833,#17834))
REPRESENTATION_CONTEXT('','3D')
);
#17830=(
GEOMETRIC_REPRESENTATION_CONTEXT(3)
GLOBAL_UNCERTAINTY_ASSIGNED_CONTEXT((#17780))
GLOBAL_UNIT_ASSIGNED_CONTEXT((#17831,#17833,#17834))
REPRESENTATION_CONTEXT('','3D')
);
#17831=(
LENGTH_UNIT()
NAMED_UNIT(*)
SI_UNIT(.CENTI.,.METRE.)
);
#17833=(
NAMED_UNIT(*)
PLANE_ANGLE_UNIT()
SI_UNIT($,.RADIAN.)
);
#17834=(
NAMED_UNIT(*)
SI_UNIT($,.STERADIAN.)
SOLID_ANGLE_UNIT()
);
#17857=SHAPE_DEFINITION_REPRESENTATION(#17906,#18028);
#17906=PRODUCT_DEFINITION_SHAPE('',$,#18078);
#18028=SHAPE_REPRESENTATION('',(#9934),#17803);
#18055=PRODUCT_DEFINITION_CONTEXT('part definition',#18204,'design');
#18078=PRODUCT_DEFINITION('Cage','Cage',#18127,#18055);
#18127=PRODUCT_DEFINITION_FORMATION('',$,#18228);
#18204=APPLICATION_CONTEXT(
'Core Data for Automotive Mechanical Design Process');
#18205=PRODUCT_CONTEXT('part definition',#18204,'mechanical');
#18228=PRODUCT('Cage','Cage','Cage',(#18205));
#18311=COLOUR_RGB('Grey',0.48,0.52,0.57);
#18312=FILL_AREA_STYLE_COLOUR('',#18311);
#18313=FILL_AREA_STYLE('',(#18312));
#18314=SURFACE_STYLE_FILL_AREA(#18313);
#18315=SURFACE_SIDE_STYLE('',(#18314));
#18316=SURFACE_STYLE_USAGE(.BOTH.,#18315);
#18317=PRESENTATION_STYLE_ASSIGNMENT((#18316));
ENDSEC;
END-ISO-10303-21;
